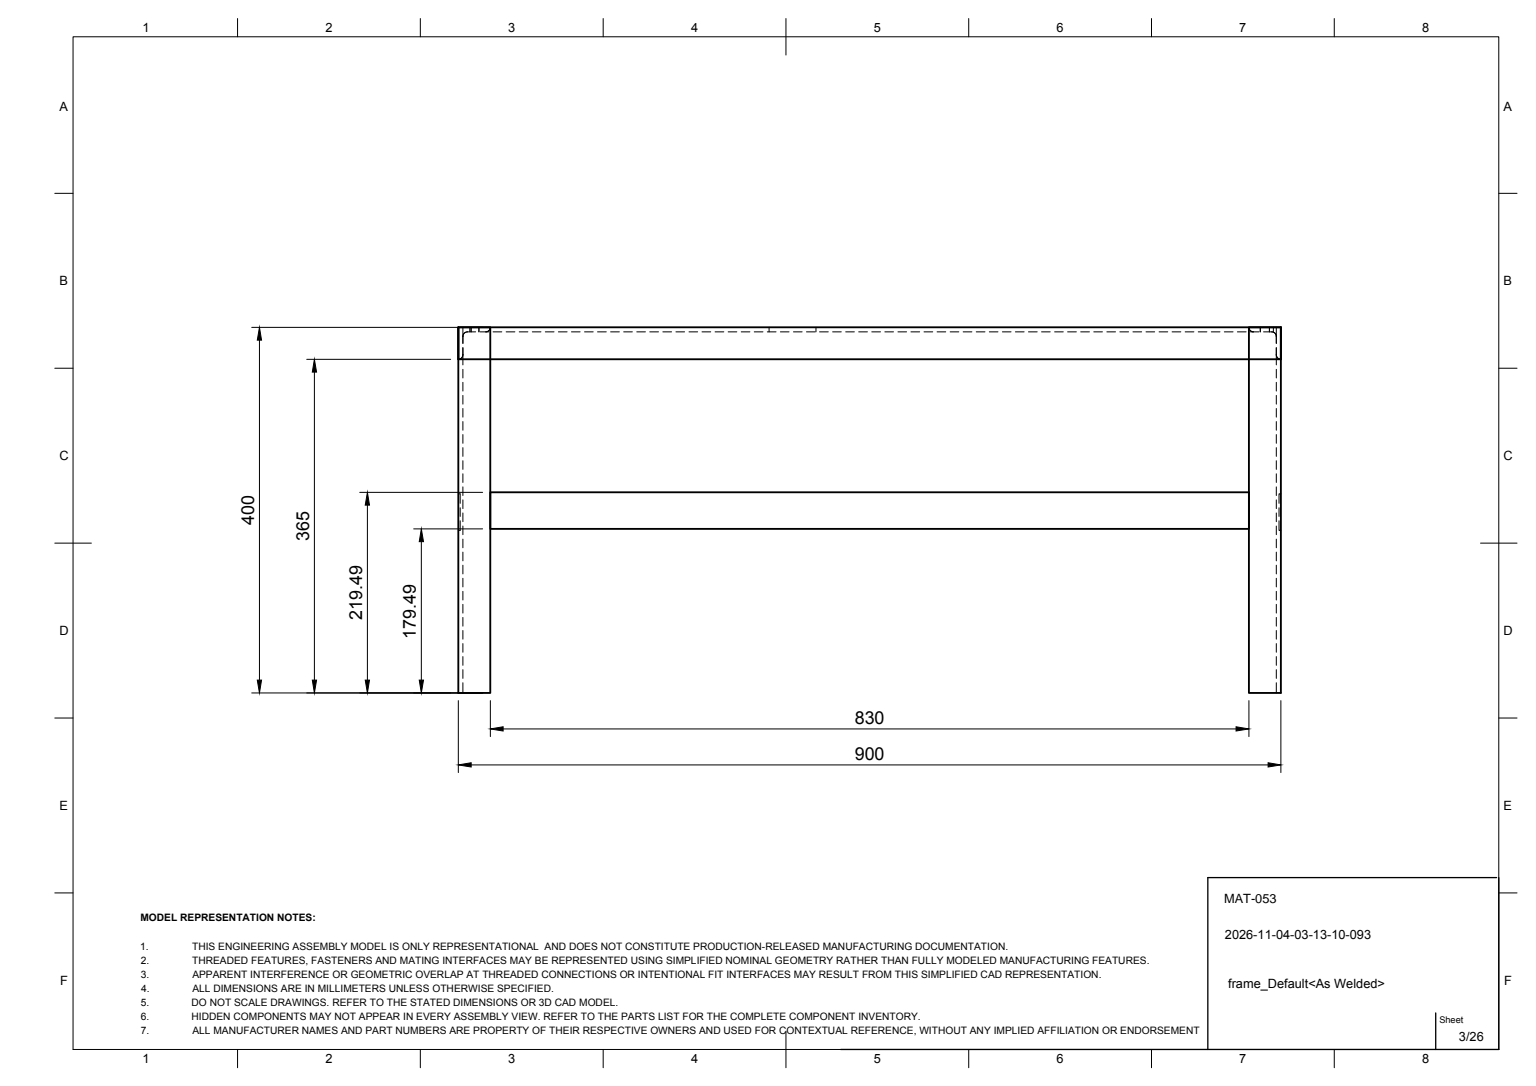
ISO-10303-21;
HEADER;
FILE_DESCRIPTION (('STEP AP214'),
    '1' );
FILE_NAME ('frame_Default<As Welded>.step',
    '2026-10-10T03:43:58',
    ( '' ),
    ( '' ),
    'SwSTEP 2.0',
    'SolidWorks 2026',
    '' );
FILE_SCHEMA (( 'AUTOMOTIVE_DESIGN' ));
ENDSEC;

DATA;
#18=ORIENTED_EDGE ( 'NONE', *, *, #43591, .T. ) ;
#28=DIRECTION ( 'NONE',  ( -1.000000000000000000, -1.850550996349095901E-16, -1.228197773518735191E-20 ) ) ;
#41=DIRECTION ( 'NONE',  ( -1.001915251000354105E-14, 1.000000000000000000, 5.551115123135531297E-17 ) ) ;
#49=CARTESIAN_POINT ( 'NONE',  ( 447.3372781065085633, 399.9999999999998863, 113.5502958579881891 ) ) ;
#135=VERTEX_POINT ( 'NONE', #41824 ) ;
#162=CARTESIAN_POINT ( 'NONE',  ( -444.4229916354184979, 394.6798985497181889, -128.9497041420121093 ) ) ;
#207=AXIS2_PLACEMENT_3D ( 'NONE', #62081, #45913, #12874 ) ;
#228=ORIENTED_EDGE ( 'NONE', *, *, #68309, .F. ) ;
#239=ORIENTED_EDGE ( 'NONE', *, *, #49975, .T. ) ;
#260=LINE ( 'NONE', #68864, #29041 ) ;
#261=VECTOR ( 'NONE', #60433, 1000.000000000000000 ) ;
#278=ORIENTED_EDGE ( 'NONE', *, *, #36224, .T. ) ;
#299=DIRECTION ( 'NONE',  ( 1.000000000000000000, 1.024558601614476894E-14, -9.899298618516476860E-15 ) ) ;
#301=VECTOR ( 'NONE', #7610, 1000.000000000000000 ) ;
#320=CARTESIAN_POINT ( 'NONE',  ( 442.3372781065083359, 370.0000000000043201, 108.5502958579838833 ) ) ;
#323=DIRECTION ( 'NONE',  ( 0.000000000000000000, 0.000000000000000000, -1.000000000000000000 ) ) ;
#329=FACE_OUTER_BOUND ( 'NONE', #61642, .T. ) ;
#352=DIRECTION ( 'NONE',  ( -0.7071067811865543451, -7.105427357601001070E-15, -0.7071067811865408004 ) ) ;
#366=VERTEX_POINT ( 'NONE', #38615 ) ;
#379=CYLINDRICAL_SURFACE ( 'NONE', #33876, 5.000000000000170530 ) ;
#403=AXIS2_PLACEMENT_3D ( 'NONE', #39353, #38653, #43213 ) ;
#416=CIRCLE ( 'NONE', #39744, 5.000000000000004441 ) ;
#423=AXIS2_PLACEMENT_3D ( 'NONE', #15656, #48667, #10364 ) ;
#492=CARTESIAN_POINT ( 'NONE',  ( -417.6627218934913230, 179.4906275429376308, 113.5502958579881749 ) ) ;
#493=DIRECTION ( 'NONE',  ( -2.921639538487254261E-16, -1.134144525784205431E-35, -1.000000000000000000 ) ) ;
#499=DIRECTION ( 'NONE',  ( 1.000000000000000000, 0.000000000000000000, 0.000000000000000000 ) ) ;
#500=ORIENTED_EDGE ( 'NONE', *, *, #39553, .F. ) ;
#508=DIRECTION ( 'NONE',  ( 1.000000000000000000, 0.000000000000000000, 0.000000000000000000 ) ) ;
#534=EDGE_CURVE ( 'NONE', #34523, #68707, #2552, .T. ) ;
#537=ORIENTED_EDGE ( 'NONE', *, *, #20232, .T. ) ;
#540=CARTESIAN_POINT ( 'NONE',  ( -442.6627218934913230, 1.665334536937734811E-13, 108.5502958579881749 ) ) ;
#568=VECTOR ( 'NONE', #4706, 1000.000000000000000 ) ;
#572=AXIS2_PLACEMENT_3D ( 'NONE', #9018, #25882, #35396 ) ;
#585=CARTESIAN_POINT ( 'NONE',  ( -422.6627218934914936, 399.9999999999998863, -141.4497041420118535 ) ) ;
#595=CARTESIAN_POINT ( 'NONE',  ( 107.3013380801408800, 395.0000000000065938, -128.9497041420121093 ) ) ;
#640=ADVANCED_FACE ( 'NONE', ( #57916 ), #9734, .T. ) ;
#646=CARTESIAN_POINT ( 'NONE',  ( 447.3372781065089612, 365.0000000000064233, -146.4497041420121377 ) ) ;
#648=ORIENTED_EDGE ( 'NONE', *, *, #3366, .T. ) ;
#665=FACE_OUTER_BOUND ( 'NONE', #60065, .T. ) ;
#678=CARTESIAN_POINT ( 'NONE',  ( 414.4083459183740388, 395.0000000000000568, -113.5207719538772579 ) ) ;
#699=CARTESIAN_POINT ( 'NONE',  ( 447.3372781065085633, 400.0000000000000568, -116.4497041420118393 ) ) ;
#723=CARTESIAN_POINT ( 'NONE',  ( -442.6627218934912662, 394.9999999999998295, 113.5502958579881465 ) ) ;
#726=ORIENTED_EDGE ( 'NONE', *, *, #5061, .T. ) ;
#732=CARTESIAN_POINT ( 'NONE',  ( -445.5916540816263591, 395.0000000000064801, -139.3786363301466906 ) ) ;
#742=ORIENTED_EDGE ( 'NONE', *, *, #24252, .T. ) ;
#756=AXIS2_PLACEMENT_3D ( 'NONE', #20145, #23779, #63754 ) ;
#768=ADVANCED_FACE ( 'NONE', ( #22611 ), #7498, .F. ) ;
#788=EDGE_CURVE ( 'NONE', #34907, #36914, #33986, .T. ) ;
#795=CARTESIAN_POINT ( 'NONE',  ( 412.3372781065085633, 219.4906275429376308, 113.5502958579881749 ) ) ;
#803=DIRECTION ( 'NONE',  ( -0.7071067811865405783, -7.105427357601001070E-15, 0.7071067811865545671 ) ) ;
#804=ORIENTED_EDGE ( 'NONE', *, *, #57601, .F. ) ;
#807=LINE ( 'NONE', #22262, #23012 ) ;
#810=ORIENTED_EDGE ( 'NONE', *, *, #68485, .F. ) ;
#817=EDGE_CURVE ( 'NONE', #39831, #41874, #11117, .T. ) ;
#829=ORIENTED_EDGE ( 'NONE', *, *, #20982, .F. ) ;
#869=CARTESIAN_POINT ( 'NONE',  ( -444.2280788262714282, 394.7493581867591388, -130.3782898954363532 ) ) ;
#876=EDGE_CURVE ( 'NONE', #55579, #9108, #39602, .T. ) ;
#907=AXIS2_PLACEMENT_3D ( 'NONE', #46556, #43247, #32374 ) ;
#910=VERTEX_POINT ( 'NONE', #6888 ) ;
#929=DIRECTION ( 'NONE',  ( 1.110223024625156540E-16, 1.358505038629840220E-33, 1.000000000000000000 ) ) ;
#957=FACE_OUTER_BOUND ( 'NONE', #48813, .T. ) ;
#966=DIRECTION ( 'NONE',  ( -1.000000000000000000, 0.000000000000000000, 0.000000000000000000 ) ) ;
#979=ORIENTED_EDGE ( 'NONE', *, *, #14468, .F. ) ;
#983=LINE ( 'NONE', #36278, #21334 ) ;
#1010=FACE_OUTER_BOUND ( 'NONE', #37761, .T. ) ;
#1019=DIRECTION ( 'NONE',  ( -1.000000000000000000, 0.000000000000000000, 0.000000000000000000 ) ) ;
#1062=FACE_OUTER_BOUND ( 'NONE', #64312, .T. ) ;
#1077=ORIENTED_EDGE ( 'NONE', *, *, #16773, .T. ) ;
#1078=CARTESIAN_POINT ( 'NONE',  ( -447.6627218934918346, 392.9289321881408910, -141.4497041420121661 ) ) ;
#1084=CYLINDRICAL_SURFACE ( 'NONE', #16978, 5.000000000000004441 ) ;
#1107=CARTESIAN_POINT ( 'NONE',  ( -443.8115333961470128, 394.8687311169578606, 93.62756966056487329 ) ) ;
#1126=LINE ( 'NONE', #65145, #9413 ) ;
#1128=DIRECTION ( 'NONE',  ( -1.000000000000000000, 1.232595164407830946E-32, 7.703719777548943412E-34 ) ) ;
#1133=CARTESIAN_POINT ( 'NONE',  ( -447.6627218934914367, 399.9999999999998863, -136.4497041420118251 ) ) ;
#1158=AXIS2_PLACEMENT_3D ( 'NONE', #24010, #19073, #25057 ) ;
#1160=DIRECTION ( 'NONE',  ( 1.232595164407830946E-32, 1.000000000000000000, 3.469446951953615421E-17 ) ) ;
#1222=CARTESIAN_POINT ( 'NONE',  ( 2.337278106504167230, 395.0000000000000000, -341.4497041420117966 ) ) ;
#1242=VECTOR ( 'NONE', #52232, 1000.000000000000000 ) ;
#1247=ORIENTED_EDGE ( 'NONE', *, *, #46850, .F. ) ;
#1264=DIRECTION ( 'NONE',  ( -3.081487911019579554E-32, -1.000000000000000000, -3.469446951953612956E-17 ) ) ;
#1275=LINE ( 'NONE', #22730, #301 ) ;
#1299=ORIENTED_EDGE ( 'NONE', *, *, #69235, .F. ) ;
#1342=CARTESIAN_POINT ( 'NONE',  ( 112.3013380801408658, 400.0000000000066507, -123.9497041420121235 ) ) ;
#1352=EDGE_CURVE ( 'NONE', #21613, #62663, #64860, .T. ) ;
#1391=ORIENTED_EDGE ( 'NONE', *, *, #21130, .F. ) ;
#1405=CARTESIAN_POINT ( 'NONE',  ( 442.3372781065085633, 399.9999999999998863, 103.5502958579881891 ) ) ;
#1409=ADVANCED_FACE ( 'NONE', ( #62002 ), #51117, .T. ) ;
#1411=EDGE_CURVE ( 'NONE', #51862, #23473, #29508, .T. ) ;
#1422=VECTOR ( 'NONE', #58262, 1000.000000000000000 ) ;
#1465=ORIENTED_EDGE ( 'NONE', *, *, #37162, .F. ) ;
#1521=VECTOR ( 'NONE', #55884, 1000.000000000000000 ) ;
#1538=VECTOR ( 'NONE', #21960, 1000.000000000000000 ) ;
#1541=CARTESIAN_POINT ( 'NONE',  ( -422.6627218934913230, 399.9999999999997726, 108.5502958579881891 ) ) ;
#1552=UNCERTAINTY_MEASURE_WITH_UNIT (LENGTH_MEASURE( 1.000000000000000082E-05 ), #45317, 'distance_accuracy_value', 'NONE');
#1580=VERTEX_POINT ( 'NONE', #18236 ) ;
#1591=LINE ( 'NONE', #17777, #28115 ) ;
#1592=LINE ( 'NONE', #44135, #22665 ) ;
#1640=DIRECTION ( 'NONE',  ( 1.850371928290090422E-16, -1.000000000000000000, -1.110223024625156171E-16 ) ) ;
#1652=EDGE_CURVE ( 'NONE', #46890, #13975, #15383, .T. ) ;
#1660=ORIENTED_EDGE ( 'NONE', *, *, #34022, .F. ) ;
#1666=EDGE_CURVE ( 'NONE', #1887, #55194, #16064, .T. ) ;
#1687=ADVANCED_FACE ( 'NONE', ( #31557 ), #48747, .F. ) ;
#1736=CARTESIAN_POINT ( 'NONE',  ( -20.16272189348855903, 400.0000000000064801, 321.0502958579853043 ) ) ;
#1748=DIRECTION ( 'NONE',  ( 0.000000000000000000, -1.000000000000000000, 0.000000000000000000 ) ) ;
#1776=CIRCLE ( 'NONE', #53407, 5.000000000000170530 ) ;
#1784=VERTEX_POINT ( 'NONE', #38561 ) ;
#1786=EDGE_CURVE ( 'NONE', #2896, #55220, #18505, .T. ) ;
#1787=CARTESIAN_POINT ( 'NONE',  ( -447.6627218934913230, 399.9999999999997726, 83.55029585798818914 ) ) ;
#1788=AXIS2_PLACEMENT_3D ( 'NONE', #24721, #40533, #2565 ) ;
#1808=FACE_OUTER_BOUND ( 'NONE', #63947, .T. ) ;
#1827=CARTESIAN_POINT ( 'NONE',  ( 445.3372781065085633, 177.8591479523844612, -111.4497041420119388 ) ) ;
#1838=VECTOR ( 'NONE', #46198, 1000.000000000000000 ) ;
#1849=AXIS2_PLACEMENT_3D ( 'NONE', #48486, #323, #32687 ) ;
#1868=ORIENTED_EDGE ( 'NONE', *, *, #4757, .T. ) ;
#1882=CARTESIAN_POINT ( 'NONE',  ( 447.3372781065085633, 217.8591479523844612, -111.4497041420119388 ) ) ;
#1887=VERTEX_POINT ( 'NONE', #41685 ) ;
#1891=FACE_OUTER_BOUND ( 'NONE', #33481, .T. ) ;
#1918=CARTESIAN_POINT ( 'NONE',  ( 112.3013380801408658, 388.0000000000065938, -123.9497041420121235 ) ) ;
#1981=ORIENTED_EDGE ( 'NONE', *, *, #63831, .F. ) ;
#1996=EDGE_CURVE ( 'NONE', #60543, #5635, #11609, .T. ) ;
#2025=FACE_OUTER_BOUND ( 'NONE', #12896, .T. ) ;
#2053=EDGE_CURVE ( 'NONE', #43634, #38637, #20566, .T. ) ;
#2108=CARTESIAN_POINT ( 'NONE',  ( 424.8372781065087906, 400.0000000000067075, -123.9497041420121235 ) ) ;
#2130=( GEOMETRIC_REPRESENTATION_CONTEXT ( 3 ) GLOBAL_UNCERTAINTY_ASSIGNED_CONTEXT ( ( #8581 ) ) GLOBAL_UNIT_ASSIGNED_CONTEXT ( ( #28794, #2407, #61144 ) ) REPRESENTATION_CONTEXT ( 'NONE', 'WORKASPACE' ) );
#2145=EDGE_LOOP ( 'NONE', ( #5278, #8405, #51535 ) ) ;
#2147=CARTESIAN_POINT ( 'NONE',  ( -442.6627218934916641, 394.9999999999954525, 103.5502958579924808 ) ) ;
#2180=ORIENTED_EDGE ( 'NONE', *, *, #21990, .T. ) ;
#2250=AXIS2_PLACEMENT_3D ( 'NONE', #44344, #38734, #56292 ) ;
#2260=DIRECTION ( 'NONE',  ( 0.000000000000000000, 1.000000000000000000, 0.000000000000000000 ) ) ;
#2295=DIRECTION ( 'NONE',  ( -1.000000000000000000, 0.000000000000000000, 0.000000000000000000 ) ) ;
#2296=CARTESIAN_POINT ( 'NONE',  ( 445.3372781065086201, 177.8591479523844612, 78.55029585798806124 ) ) ;
#2306=EDGE_CURVE ( 'NONE', #4870, #42101, #55269, .T. ) ;
#2311=ORIENTED_EDGE ( 'NONE', *, *, #31125, .T. ) ;
#2325=ORIENTED_EDGE ( 'NONE', *, *, #51865, .F. ) ;
#2331=PLANE ( 'NONE',  #41598 ) ;
#2335=ORIENTED_EDGE ( 'NONE', *, *, #23615, .F. ) ;
#2342=LINE ( 'NONE', #66717, #52285 ) ;
#2350=SHAPE_REPRESENTATION_RELATIONSHIP ( 'NONE' , 'NONE' ,  #2894, #64275 ) ;
#2405=STYLED_ITEM ( 'NONE', ( #35553 ), #16744 ) ;
#2406=DIRECTION ( 'NONE',  ( -4.270088556250601699E-16, -0.000000000000000000, -1.000000000000000000 ) ) ;
#2407=( NAMED_UNIT ( * ) PLANE_ANGLE_UNIT ( ) SI_UNIT ( $, .RADIAN. ) );
#2464=EDGE_LOOP ( 'NONE', ( #43968, #36978, #53446, #55906, #66488, #18902, #35917 ) ) ;
#2487=ADVANCED_FACE ( 'NONE', ( #5266 ), #48156, .T. ) ;
#2503=DIRECTION ( 'NONE',  ( 1.387778780781446169E-16, -1.000000000000000000, -3.469446951953615421E-17 ) ) ;
#2532=CARTESIAN_POINT ( 'NONE',  ( -417.6627218934913799, 399.9999999999998295, -111.4497041420118251 ) ) ;
#2536=CARTESIAN_POINT ( 'NONE',  ( -444.4229916354184979, 394.6798985497181320, 96.05029585798874336 ) ) ;
#2552=CIRCLE ( 'NONE', #39606, 5.000000000000004441 ) ;
#2565=DIRECTION ( 'NONE',  ( 1.000000000000000000, -9.109522253334613014E-16, 0.000000000000000000 ) ) ;
#2568=EDGE_CURVE ( 'NONE', #37758, #24336, #57705, .T. ) ;
#2583=ORIENTED_EDGE ( 'NONE', *, *, #50107, .F. ) ;
#2595=VECTOR ( 'NONE', #6924, 1000.000000000000000 ) ;
#2601=AXIS2_PLACEMENT_3D ( 'NONE', #24393, #62712, #45834 ) ;
#2604=ORIENTED_EDGE ( 'NONE', *, *, #10155, .T. ) ;
#2622=DIRECTION ( 'NONE',  ( 1.000000000000000000, 0.000000000000000000, 0.000000000000000000 ) ) ;
#2624=CARTESIAN_POINT ( 'NONE',  ( -452.6627218934912662, 364.9999999999998863, 113.5502958579877912 ) ) ;
#2681=LINE ( 'NONE', #55439, #22046 ) ;
#2713=EDGE_LOOP ( 'NONE', ( #26660, #62305, #27434, #31457 ) ) ;
#2752=FACE_OUTER_BOUND ( 'NONE', #52532, .T. ) ;
#2761=( NAMED_UNIT ( * ) PLANE_ANGLE_UNIT ( ) SI_UNIT ( $, .RADIAN. ) );
#2765=CARTESIAN_POINT ( 'NONE',  ( 112.3013380801407095, 388.0000000000077307, 91.05029585798746439 ) ) ;
#2771=CARTESIAN_POINT ( 'NONE',  ( -452.6627218934912094, 399.9999999999998295, 113.5502958579882602 ) ) ;
#2791=CARTESIAN_POINT ( 'NONE',  ( -452.6627218934913230, 399.9999999999997726, 78.55029585798818914 ) ) ;
#2833=PLANE ( 'NONE',  #68014 ) ;
#2834=VECTOR ( 'NONE', #1264, 1000.000000000000000 ) ;
#2838=CARTESIAN_POINT ( 'NONE',  ( 412.3372781065085633, 219.4906275429376308, 111.5502958579881749 ) ) ;
#2857=VERTEX_POINT ( 'NONE', #66811 ) ;
#2884=EDGE_CURVE ( 'NONE', #36808, #910, #34790, .T. ) ;
#2891=VECTOR ( 'NONE', #10003, 1000.000000000000000 ) ;
#2894=SHAPE_REPRESENTATION ( 'frame_Default<As Welded>', ( #66832 ), #12890 ) ;
#2896=VERTEX_POINT ( 'NONE', #68432 ) ;
#2914=ORIENTED_EDGE ( 'NONE', *, *, #9847, .T. ) ;
#2925=CARTESIAN_POINT ( 'NONE',  ( -450.6627218934913230, 217.8591479523843475, 78.55029585798814651 ) ) ;
#2948=EDGE_CURVE ( 'NONE', #44967, #17356, #65568, .T. ) ;
#2953=EDGE_CURVE ( 'NONE', #6937, #46890, #35233, .T. ) ;
#2955=EDGE_CURVE ( 'NONE', #36796, #51074, #58217, .T. ) ;
#2956=CARTESIAN_POINT ( 'NONE',  ( -439.4229916354183274, 400.0000000000064801, 96.05029585798874336 ) ) ;
#2958=CARTESIAN_POINT ( 'NONE',  ( 437.3372781065085633, 390.0000000000001137, -146.4497041420117966 ) ) ;
#2979=DIRECTION ( 'NONE',  ( -1.387778780781445922E-16, 1.000000000000000000, 1.232595164407830946E-32 ) ) ;
#2980=DIRECTION ( 'NONE',  ( 9.729495617646301779E-15, -5.551115123125782702E-17, 1.000000000000000000 ) ) ;
#2982=VECTOR ( 'NONE', #47038, 1000.000000000000000 ) ;
#2983=ORIENTED_EDGE ( 'NONE', *, *, #34114, .F. ) ;
#2985=DIRECTION ( 'NONE',  ( -1.000000000000000000, 0.000000000000000000, 0.000000000000000000 ) ) ;
#3011=DIRECTION ( 'NONE',  ( -1.000000000000000000, 0.000000000000000000, 0.000000000000000000 ) ) ;
#3038=AXIS2_PLACEMENT_3D ( 'NONE', #5533, #54754, #23111 ) ;
#3044=EDGE_LOOP ( 'NONE', ( #2914, #25695, #29990, #1660 ) ) ;
#3057=PLANE ( 'NONE',  #30957 ) ;
#3091=AXIS2_PLACEMENT_3D ( 'NONE', #61680, #34958, #66297 ) ;
#3096=EDGE_CURVE ( 'NONE', #32147, #11742, #65456, .T. ) ;
#3100=ORIENTED_EDGE ( 'NONE', *, *, #817, .T. ) ;
#3113=VERTEX_POINT ( 'NONE', #34963 ) ;
#3116=ADVANCED_FACE ( 'NONE', ( #51138 ), #14198, .T. ) ;
#3120=CARTESIAN_POINT ( 'NONE',  ( -452.6627218934918346, 365.0000000000064233, -146.4497041420121377 ) ) ;
#3122=( NAMED_UNIT ( * ) PLANE_ANGLE_UNIT ( ) SI_UNIT ( $, .RADIAN. ) );
#3151=ADVANCED_FACE ( 'NONE', ( #51491 ), #25107, .T. ) ;
#3161=VERTEX_POINT ( 'NONE', #9956 ) ;
#3167=ORIENTED_EDGE ( 'NONE', *, *, #33592, .T. ) ;
#3207=CARTESIAN_POINT ( 'NONE',  ( 442.3372781065085633, 400.0000000000000568, -116.4497041420118393 ) ) ;
#3224=CARTESIAN_POINT ( 'NONE',  ( 437.3372781065085633, 399.9999999999998863, 103.5502958579881891 ) ) ;
#3237=AXIS2_PLACEMENT_3D ( 'NONE', #6631, #26704, #65382 ) ;
#3240=CARTESIAN_POINT ( 'NONE',  ( 417.3372781065086770, 0.000000000000000000, 108.5502958579881891 ) ) ;
#3251=CARTESIAN_POINT ( 'NONE',  ( -417.6627218934913230, 219.4906275429376308, -146.4497041420118819 ) ) ;
#3257=EDGE_CURVE ( 'NONE', #19058, #41538, #58468, .T. ) ;
#3264=EDGE_LOOP ( 'NONE', ( #28641, #52255, #19541, #43229, #54328, #3932, #7134, #33574, #55209, #62511, #15106, #27197 ) ) ;
#3289=LINE ( 'NONE', #24747, #33740 ) ;
#3298=CARTESIAN_POINT ( 'NONE',  ( 437.3372781065085633, 395.0000000000001137, -146.4497041420117966 ) ) ;
#3304=CARTESIAN_POINT ( 'NONE',  ( 412.3372781065085633, 219.4906275429376308, 113.5502958579881749 ) ) ;
#3316=FACE_OUTER_BOUND ( 'NONE', #58462, .T. ) ;
#3319=ORIENTED_EDGE ( 'NONE', *, *, #44714, .T. ) ;
#3338=DIRECTION ( 'NONE',  ( 0.000000000000000000, 6.123233995736761105E-17, -1.000000000000000000 ) ) ;
#3362=AXIS2_PLACEMENT_3D ( 'NONE', #53763, #27037, #48468 ) ;
#3366=EDGE_CURVE ( 'NONE', #60705, #17566, #50001, .T. ) ;
#3371=VERTEX_POINT ( 'NONE', #54575 ) ;
#3393=CARTESIAN_POINT ( 'NONE',  ( -447.6627218934919483, 370.0000000000056275, -141.4497041420121661 ) ) ;
#3394=CARTESIAN_POINT ( 'NONE',  ( 14.83727810650406731, 400.0000000000001137, -353.9497041420119672 ) ) ;
#3400=ORIENTED_EDGE ( 'NONE', *, *, #22879, .F. ) ;
#3414=ORIENTED_EDGE ( 'NONE', *, *, #12766, .T. ) ;
#3424=EDGE_LOOP ( 'NONE', ( #40584, #35783, #60824, #8916 ) ) ;
#3438=PLANE ( 'NONE',  #44136 ) ;
#3450=ORIENTED_EDGE ( 'NONE', *, *, #23507, .T. ) ;
#3458=CARTESIAN_POINT ( 'NONE',  ( -452.6627218934913799, 364.9999999999998295, -146.4497041420117966 ) ) ;
#3460=AXIS2_PLACEMENT_3D ( 'NONE', #7707, #40739, #29155 ) ;
#3481=CARTESIAN_POINT ( 'NONE',  ( 447.3372781065086201, 0.000000000000000000, 83.55029585798817493 ) ) ;
#3487=DIRECTION ( 'NONE',  ( 1.387778780781445429E-16, -1.000000000000000000, -3.081487911019577365E-33 ) ) ;
#3490=VECTOR ( 'NONE', #9251, 1000.000000000000114 ) ;
#3534=SURFACE_SIDE_STYLE ('',( #42208 ) ) ;
#3547=VECTOR ( 'NONE', #40734, 1000.000000000000000 ) ;
#3549=DIRECTION ( 'NONE',  ( 0.7071067811865476838, 1.110223024625156294E-16, 0.7071067811865474617 ) ) ;
#3582=ORIENTED_EDGE ( 'NONE', *, *, #15343, .F. ) ;
#3586=AXIS2_PLACEMENT_3D ( 'NONE', #12327, #33447, #27444 ) ;
#3590=VECTOR ( 'NONE', #42220, 1000.000000000000000 ) ;
#3631=DIRECTION ( 'NONE',  ( 0.7071067811865474617, -5.551115123125781716E-16, 0.7071067811865475727 ) ) ;
#3632=ADVANCED_FACE ( 'NONE', ( #23511 ), #48674, .T. ) ;
#3644=EDGE_CURVE ( 'NONE', #21636, #60543, #50981, .T. ) ;
#3649=AXIS2_PLACEMENT_3D ( 'NONE', #4128, #13639, #40372 ) ;
#3651=LINE ( 'NONE', #53889, #16378 ) ;
#3702=CARTESIAN_POINT ( 'NONE',  ( 447.3372781065085633, 400.0000000000000568, -146.4497041420118251 ) ) ;
#3703=CARTESIAN_POINT ( 'NONE',  ( 412.3372781065082791, 400.0000000000040927, 78.55029585798418168 ) ) ;
#3716=ORIENTED_EDGE ( 'NONE', *, *, #64221, .T. ) ;
#3753=ADVANCED_FACE ( 'NONE', ( #59941 ), #6837, .T. ) ;
#3759=DIRECTION ( 'NONE',  ( 6.405132834375901070E-16, -1.000000000000000000, -6.405132834375902056E-16 ) ) ;
#3784=ADVANCED_FACE ( 'NONE', ( #7893 ), #49385, .T. ) ;
#3804=CARTESIAN_POINT ( 'NONE',  ( -452.6627218934914367, 399.9999999999998863, -146.4497041420118251 ) ) ;
#3849=ORIENTED_EDGE ( 'NONE', *, *, #26324, .F. ) ;
#3854=EDGE_LOOP ( 'NONE', ( #26584, #28103, #17107, #64079, #38779, #9643, #4054 ) ) ;
#3867=EDGE_LOOP ( 'NONE', ( #36108, #28405, #537, #61706 ) ) ;
#3892=DIRECTION ( 'NONE',  ( 0.000000000000000000, -6.123233995736762338E-17, 1.000000000000000000 ) ) ;
#3904=LINE ( 'NONE', #29250, #45362 ) ;
#3929=ORIENTED_EDGE ( 'NONE', *, *, #39789, .T. ) ;
#3932=ORIENTED_EDGE ( 'NONE', *, *, #3096, .T. ) ;
#3959=EDGE_CURVE ( 'NONE', #38702, #53656, #25115, .T. ) ;
#3963=ORIENTED_EDGE ( 'NONE', *, *, #8078, .F. ) ;
#4033=ORIENTED_EDGE ( 'NONE', *, *, #59864, .T. ) ;
#4050=ADVANCED_FACE ( 'NONE', ( #31754 ), #69386, .T. ) ;
#4054=ORIENTED_EDGE ( 'NONE', *, *, #64477, .F. ) ;
#4055=DIRECTION ( 'NONE',  ( -1.000000000000000000, 1.540743955509788682E-33, 1.110223024625156540E-16 ) ) ;
#4098=ORIENTED_EDGE ( 'NONE', *, *, #66400, .T. ) ;
#4118=EDGE_LOOP ( 'NONE', ( #27509, #50059, #51468, #64476, #63468, #11482, #54903 ) ) ;
#4128=CARTESIAN_POINT ( 'NONE',  ( -422.6627218934914367, 0.000000000000000000, -146.4497041420118251 ) ) ;
#4132=ADVANCED_FACE ( 'NONE', ( #15922 ), #15236, .T. ) ;
#4156=CARTESIAN_POINT ( 'NONE',  ( -449.7337897053568554, 364.9999999999998295, -143.5207719538772722 ) ) ;
#4159=ORIENTED_EDGE ( 'NONE', *, *, #52250, .F. ) ;
#4203=CARTESIAN_POINT ( 'NONE',  ( 437.3372781065085633, 394.9999999999999432, 91.05029585798857283 ) ) ;
#4214=CARTESIAN_POINT ( 'NONE',  ( 412.3372781065085633, 219.4906275429376308, -144.4497041420117682 ) ) ;
#4215=VERTEX_POINT ( 'NONE', #29594 ) ;
#4254=DIRECTION ( 'NONE',  ( 1.387778780781445922E-16, -1.000000000000000000, -1.232595164407830946E-32 ) ) ;
#4271=EDGE_LOOP ( 'NONE', ( #40131, #56927, #23005, #48343 ) ) ;
#4293=VECTOR ( 'NONE', #68342, 1000.000000000000000 ) ;
#4319=CARTESIAN_POINT ( 'NONE',  ( 445.3372781065086201, 177.8591479523844612, 78.55029585798806124 ) ) ;
#4339=( GEOMETRIC_REPRESENTATION_CONTEXT ( 3 ) GLOBAL_UNCERTAINTY_ASSIGNED_CONTEXT ( ( #9258 ) ) GLOBAL_UNIT_ASSIGNED_CONTEXT ( ( #38027, #66523, #46082 ) ) REPRESENTATION_CONTEXT ( 'NONE', 'WORKASPACE' ) );
#4340=DIRECTION ( 'NONE',  ( -4.946224812893509176E-48, 1.000000000000000000, 3.697785493223491743E-32 ) ) ;
#4348=EDGE_LOOP ( 'NONE', ( #4033, #62830, #17819, #64317 ) ) ;
#4384=AXIS2_PLACEMENT_3D ( 'NONE', #3481, #29873, #67509 ) ;
#4395=CARTESIAN_POINT ( 'NONE',  ( -417.6627218934913230, 219.4906275429376308, 111.5502958579881749 ) ) ;
#4400=DIRECTION ( 'NONE',  ( -3.946780934433987212E-15, -1.000000000000000000, 5.551115123125782702E-17 ) ) ;
#4404=VERTEX_POINT ( 'NONE', #67182 ) ;
#4450=DIRECTION ( 'NONE',  ( -0.7071067811865543451, -7.105427357601001070E-15, -0.7071067811865408004 ) ) ;
#4458=ADVANCED_FACE ( 'NONE', ( #43861 ), #27341, .T. ) ;
#4492=CARTESIAN_POINT ( 'NONE',  ( 437.3372781065086201, 0.000000000000000000, -141.4497041420118251 ) ) ;
#4507=ORIENTED_EDGE ( 'NONE', *, *, #67988, .F. ) ;
#4515=DIRECTION ( 'NONE',  ( 0.7071067811865475727, 0.000000000000000000, 0.7071067811865474617 ) ) ;
#4564=DIRECTION ( 'NONE',  ( 1.000000000000000000, 3.697785493223491743E-32, 0.000000000000000000 ) ) ;
#4617=EDGE_CURVE ( 'NONE', #55210, #15602, #36710, .T. ) ;
#4632=LINE ( 'NONE', #15196, #49150 ) ;
#4649=SURFACE_STYLE_USAGE ( .BOTH. , #58450 ) ;
#4650=PLANE ( 'NONE',  #24544 ) ;
#4654=EDGE_CURVE ( 'NONE', #23082, #15354, #60817, .T. ) ;
#4675=VERTEX_POINT ( 'NONE', #37729 ) ;
#4691=COLOUR_RGB ( '',0.7921568627450980005, 0.8196078431372548767, 0.9333333333333333481 ) ;
#4706=DIRECTION ( 'NONE',  ( 0.000000000000000000, -1.000000000000000000, 1.479221584281239571E-31 ) ) ;
#4708=ORIENTED_EDGE ( 'NONE', *, *, #14752, .F. ) ;
#4757=EDGE_CURVE ( 'NONE', #38637, #41110, #62186, .T. ) ;
#4775=VERTEX_POINT ( 'NONE', #2536 ) ;
#4811=LINE ( 'NONE', #15720, #2982 ) ;
#4836=EDGE_LOOP ( 'NONE', ( #31185, #40353, #53092, #63097 ) ) ;
#4838=FILL_AREA_STYLE_COLOUR ( '', #64366 ) ;
#4870=VERTEX_POINT ( 'NONE', #26755 ) ;
#4877=ORIENTED_EDGE ( 'NONE', *, *, #51267, .T. ) ;
#4921=ORIENTED_EDGE ( 'NONE', *, *, #14230, .T. ) ;
#4953=EDGE_LOOP ( 'NONE', ( #54643, #42832, #50469, #17326 ) ) ;
#4963=ORIENTED_EDGE ( 'NONE', *, *, #67890, .F. ) ;
#4969=CARTESIAN_POINT ( 'NONE',  ( 429.8372781065087338, 388.0000000000065938, 91.05029585798857283 ) ) ;
#4971=CARTESIAN_POINT ( 'NONE',  ( 445.3372781065085633, 177.8591479523844612, -111.4497041420119388 ) ) ;
#4988=EDGE_LOOP ( 'NONE', ( #67374, #3849, #16908, #44677, #2325, #29922, #50568 ) ) ;
#5005=ORIENTED_EDGE ( 'NONE', *, *, #30906, .T. ) ;
#5020=VECTOR ( 'NONE', #68078, 1000.000000000000000 ) ;
#5023=CARTESIAN_POINT ( 'NONE',  ( -439.4229916354183842, 388.0000000000064801, -128.9497041420121093 ) ) ;
#5031=AXIS2_PLACEMENT_3D ( 'NONE', #48409, #43149, #64619 ) ;
#5050=EDGE_CURVE ( 'NONE', #55210, #28296, #17940, .T. ) ;
#5061=EDGE_CURVE ( 'NONE', #67779, #9014, #65792, .T. ) ;
#5064=DIRECTION ( 'NONE',  ( -1.000000000000000000, 0.000000000000000000, -1.110223024625156294E-16 ) ) ;
#5084=ORIENTED_EDGE ( 'NONE', *, *, #25971, .T. ) ;
#5101=DIRECTION ( 'NONE',  ( 1.000000000000000000, 1.001918829714556097E-14, -9.899279560275163638E-15 ) ) ;
#5103=CARTESIAN_POINT ( 'NONE',  ( -442.6627218934913799, 0.000000000000000000, -136.4497041420118251 ) ) ;
#5135=( BOUNDED_CURVE ( )  B_SPLINE_CURVE ( 3, ( #39750, #65803, #55574, #17599 ),
 .UNSPECIFIED., .F., .F. ) 
 B_SPLINE_CURVE_WITH_KNOTS ( ( 4, 4 ),
 ( 1.570796326794883679, 3.141592653589778461 ),
 .UNSPECIFIED. ) 
 CURVE ( )  GEOMETRIC_REPRESENTATION_ITEM ( )  RATIONAL_B_SPLINE_CURVE ( ( 1.000000000000000000, 0.8047378541243654926, 0.8047378541243654926, 1.000000000000000000 ) ) 
 REPRESENTATION_ITEM ( '' )  );
#5153=DIRECTION ( 'NONE',  ( -1.000000000000000000, 0.000000000000000000, 0.000000000000000000 ) ) ;
#5187=ORIENTED_EDGE ( 'NONE', *, *, #12766, .F. ) ;
#5225=DIRECTION ( 'NONE',  ( 1.387778780781445922E-16, -1.000000000000000000, 0.000000000000000000 ) ) ;
#5228=FACE_OUTER_BOUND ( 'NONE', #4118, .T. ) ;
#5234=EDGE_CURVE ( 'NONE', #25372, #38916, #8075, .T. ) ;
#5247=SURFACE_STYLE_USAGE ( .BOTH. , #43554 ) ;
#5266=FACE_OUTER_BOUND ( 'NONE', #39432, .T. ) ;
#5278=ORIENTED_EDGE ( 'NONE', *, *, #1996, .F. ) ;
#5286=AXIS2_PLACEMENT_3D ( 'NONE', #46791, #20396, #24661 ) ;
#5302=ADVANCED_FACE ( 'NONE', ( #29524 ), #29883, .T. ) ;
#5384=CARTESIAN_POINT ( 'NONE',  ( -417.6627218934913230, 179.4906275429376308, 111.5502958579881749 ) ) ;
#5412=DIRECTION ( 'NONE',  ( 1.000000000000000000, 1.850550996349095901E-16, 1.228197773518735191E-20 ) ) ;
#5416=DIRECTION ( 'NONE',  ( -0.7071067811865473507, 6.441404958702665783E-16, 0.7071067811865477948 ) ) ;
#5448=CARTESIAN_POINT ( 'NONE',  ( -442.6627218934913799, 394.9999999999998295, -132.7581352960343679 ) ) ;
#5476=STYLED_ITEM ( 'NONE', ( #48551 ), #63846 ) ;
#5480=EDGE_LOOP ( 'NONE', ( #45183, #46394, #64906, #1077 ) ) ;
#5511=VERTEX_POINT ( 'NONE', #34038 ) ;
#5513=ORIENTED_EDGE ( 'NONE', *, *, #56243, .F. ) ;
#5533=CARTESIAN_POINT ( 'NONE',  ( 412.3372781065085633, 179.4906275429376024, 111.5502958579881749 ) ) ;
#5545=EDGE_CURVE ( 'NONE', #17804, #45879, #49845, .T. ) ;
#5564=VERTEX_POINT ( 'NONE', #55478 ) ;
#5579=EDGE_LOOP ( 'NONE', ( #67998, #13822, #65351, #59763 ) ) ;
#5593=CARTESIAN_POINT ( 'NONE',  ( -447.6627218934913799, 370.0000000000002274, -141.4497041420117966 ) ) ;
#5596=CARTESIAN_POINT ( 'NONE',  ( -422.6627218934914936, 399.9999999999998863, -141.4497041420118535 ) ) ;
#5635=VERTEX_POINT ( 'NONE', #42417 ) ;
#5642=CARTESIAN_POINT ( 'NONE',  ( 429.8372781065087338, 400.0000000000067075, -123.9497041420121235 ) ) ;
#5661=FACE_OUTER_BOUND ( 'NONE', #23819, .T. ) ;
#5663=DIRECTION ( 'NONE',  ( -1.850169831522831466E-16, 1.000000000000000000, 1.110223024625156294E-16 ) ) ;
#5693=VECTOR ( 'NONE', #9339, 999.9999999999998863 ) ;
#5702=DIRECTION ( 'NONE',  ( -1.850169831522831466E-16, 1.000000000000000000, 1.110223024625156294E-16 ) ) ;
#5731=ORIENTED_EDGE ( 'NONE', *, *, #3644, .T. ) ;
#5774=CIRCLE ( 'NONE', #15927, 5.000000000000004441 ) ;
#5806=ORIENTED_EDGE ( 'NONE', *, *, #10304, .T. ) ;
#5816=CARTESIAN_POINT ( 'NONE',  ( -417.6627218934913230, 179.4906275429376308, 113.5502958579881749 ) ) ;
#5823=VECTOR ( 'NONE', #69312, 1000.000000000000000 ) ;
#5857=CARTESIAN_POINT ( 'NONE',  ( 412.3372781065085633, 179.4906275429376024, 113.5502958579881749 ) ) ;
#5872=ORIENTED_EDGE ( 'NONE', *, *, #30906, .F. ) ;
#5915=CARTESIAN_POINT ( 'NONE',  ( -450.6627218934913230, 217.8591479523843475, 78.55029585798814651 ) ) ;
#5935=LINE ( 'NONE', #43575, #29982 ) ;
#5952=EDGE_CURVE ( 'NONE', #6104, #67779, #27617, .T. ) ;
#5966=FACE_OUTER_BOUND ( 'NONE', #56010, .T. ) ;
#5979=CIRCLE ( 'NONE', #21708, 5.000000000000004441 ) ;
#5994=LINE ( 'NONE', #36987, #7817 ) ;
#6017=VERTEX_POINT ( 'NONE', #40958 ) ;
#6037=VECTOR ( 'NONE', #41872, 1000.000000000000000 ) ;
#6052=LINE ( 'NONE', #54591, #30147 ) ;
#6059=CARTESIAN_POINT ( 'NONE',  ( 442.3372781065085633, 369.9999999999999432, 108.5502958579885870 ) ) ;
#6087=CYLINDRICAL_SURFACE ( 'NONE', #32050, 5.000000000000004441 ) ;
#6104=VERTEX_POINT ( 'NONE', #65088 ) ;
#6117=FACE_OUTER_BOUND ( 'NONE', #68741, .T. ) ;
#6120=DIRECTION ( 'NONE',  ( -0.7071067811865474617, 9.422489238170280455E-15, 0.7071067811865475727 ) ) ;
#6124=DIRECTION ( 'NONE',  ( 4.314083075427411048E-32, 1.000000000000000000, 6.123233995736763571E-17 ) ) ;
#6146=PLANE ( 'NONE',  #6687 ) ;
#6187=VECTOR ( 'NONE', #64225, 1000.000000000000000 ) ;
#6215=DIRECTION ( 'NONE',  ( 1.387778780781446169E-16, -1.000000000000000000, -3.469446951953615421E-17 ) ) ;
#6247=CARTESIAN_POINT ( 'NONE',  ( 112.3013380801408658, 388.0000000000065938, -133.9497041420121377 ) ) ;
#6288=LINE ( 'NONE', #48826, #31905 ) ;
#6315=ORIENTED_EDGE ( 'NONE', *, *, #50891, .F. ) ;
#6342=DIRECTION ( 'NONE',  ( -4.270088556250601699E-16, -0.000000000000000000, -1.000000000000000000 ) ) ;
#6347=DIRECTION ( 'NONE',  ( -4.270088556250601699E-16, -0.000000000000000000, -1.000000000000000000 ) ) ;
#6360=ORIENTED_EDGE ( 'NONE', *, *, #47873, .F. ) ;
#6369=CARTESIAN_POINT ( 'NONE',  ( -450.6627218934913230, 177.8591479523843475, -111.4497041420117966 ) ) ;
#6379=VECTOR ( 'NONE', #25784, 1000.000000000000000 ) ;
#6427=EDGE_CURVE ( 'NONE', #50950, #65355, #5135, .T. ) ;
#6435=EDGE_CURVE ( 'NONE', #43624, #59231, #39062, .T. ) ;
#6436=VECTOR ( 'NONE', #45427, 1000.000000000000000 ) ;
#6470=LINE ( 'NONE', #27563, #69136 ) ;
#6501=EDGE_CURVE ( 'NONE', #6937, #3371, #65968, .T. ) ;
#6503=LINE ( 'NONE', #1222, #13627 ) ;
#6507=CARTESIAN_POINT ( 'NONE',  ( -417.6627218934913230, 179.4906275429376308, 111.5502958579881749 ) ) ;
#6563=ORIENTED_EDGE ( 'NONE', *, *, #33056, .F. ) ;
#6579=FACE_OUTER_BOUND ( 'NONE', #7176, .T. ) ;
#6599=CARTESIAN_POINT ( 'NONE',  ( -444.4229916354184979, 400.0000000000064801, 96.05029585798874336 ) ) ;
#6630=CARTESIAN_POINT ( 'NONE',  ( 447.3372781065085633, 399.9999999999998863, 113.5502958579882034 ) ) ;
#6631=CARTESIAN_POINT ( 'NONE',  ( 112.3013380801407521, 388.0000000000077307, 96.05029585798746439 ) ) ;
#6659=EDGE_CURVE ( 'NONE', #54476, #2896, #67975, .T. ) ;
#6662=ADVANCED_FACE ( 'NONE', ( #62473 ), #14963, .T. ) ;
#6683=CARTESIAN_POINT ( 'NONE',  ( 433.3728120124415568, 400.0000000000067075, -132.4852380479448755 ) ) ;
#6687=AXIS2_PLACEMENT_3D ( 'NONE', #17042, #33947, #27958 ) ;
#6733=AXIS2_PLACEMENT_3D ( 'NONE', #63708, #15519, #68627 ) ;
#6746=AXIS2_PLACEMENT_3D ( 'NONE', #10254, #41, #48555 ) ;
#6783=DIRECTION ( 'NONE',  ( -1.000000000000000000, -1.850474763383843014E-16, 1.697708136181793677E-16 ) ) ;
#6798=EDGE_CURVE ( 'NONE', #1784, #51862, #11794, .T. ) ;
#6807=EDGE_LOOP ( 'NONE', ( #20423, #68819, #14156, #34926 ) ) ;
#6822=EDGE_CURVE ( 'NONE', #42101, #40754, #62676, .T. ) ;
#6837=PLANE ( 'NONE',  #43037 ) ;
#6848=EDGE_CURVE ( 'NONE', #34711, #44967, #33965, .T. ) ;
#6852=AXIS2_PLACEMENT_3D ( 'NONE', #35683, #2980, #8249 ) ;
#6853=ORIENTED_EDGE ( 'NONE', *, *, #17658, .T. ) ;
#6857=VECTOR ( 'NONE', #3338, 1000.000000000000000 ) ;
#6888=CARTESIAN_POINT ( 'NONE',  ( 50.98853755884156413, 400.0000000000065938, -133.9497041420122798 ) ) ;
#6890=ORIENTED_EDGE ( 'NONE', *, *, #63616, .F. ) ;
#6891=VECTOR ( 'NONE', #43073, 1000.000000000000000 ) ;
#6906=VERTEX_POINT ( 'NONE', #12865 ) ;
#6909=DIRECTION ( 'NONE',  ( 1.387778780781446169E-16, -1.000000000000000000, -3.469446951953615421E-17 ) ) ;
#6916=CARTESIAN_POINT ( 'NONE',  ( -452.6627218934914367, 399.9999999999998863, -111.4497041420118251 ) ) ;
#6924=DIRECTION ( 'NONE',  ( 0.000000000000000000, 1.000000000000000000, -1.479221584281239571E-31 ) ) ;
#6930=ORIENTED_EDGE ( 'NONE', *, *, #17658, .F. ) ;
#6937=VERTEX_POINT ( 'NONE', #8966 ) ;
#6955=AXIS2_PLACEMENT_3D ( 'NONE', #53845, #5663, #38379 ) ;
#6971=ADVANCED_FACE ( 'NONE', ( #9304 ), #40616, .F. ) ;
#6999=VECTOR ( 'NONE', #38253, 1000.000000000000000 ) ;
#7046=DIRECTION ( 'NONE',  ( 0.000000000000000000, -6.779273404243065824E-32, 1.000000000000000000 ) ) ;
#7117=EDGE_CURVE ( 'NONE', #62102, #66740, #10329, .T. ) ;
#7134=ORIENTED_EDGE ( 'NONE', *, *, #30790, .T. ) ;
#7159=CARTESIAN_POINT ( 'NONE',  ( 417.3372781065083359, 395.0000000000041496, 83.55029585798409641 ) ) ;
#7176=EDGE_LOOP ( 'NONE', ( #35574, #21592, #8229, #16800 ) ) ;
#7180=CYLINDRICAL_SURFACE ( 'NONE', #3091, 5.000000000000004441 ) ;
#7183=CARTESIAN_POINT ( 'NONE',  ( -447.6627218934913799, 0.000000000000000000, -136.4497041420118251 ) ) ;
#7222=CARTESIAN_POINT ( 'NONE',  ( 424.8372781065087906, 400.0000000000044906, 91.05029585798442326 ) ) ;
#7228=CARTESIAN_POINT ( 'NONE',  ( -442.6627218934913799, 0.000000000000000000, -141.4497041420118251 ) ) ;
#7279=LINE ( 'NONE', #23466, #21652 ) ;
#7293=DIRECTION ( 'NONE',  ( 1.000000000000000000, -9.109522253334613014E-16, 0.000000000000000000 ) ) ;
#7312=AXIS2_PLACEMENT_3D ( 'NONE', #27017, #26344, #5225 ) ;
#7337=EDGE_CURVE ( 'NONE', #4215, #59386, #23596, .T. ) ;
#7338=SURFACE_STYLE_USAGE ( .BOTH. , #29476 ) ;
#7355=DIRECTION ( 'NONE',  ( -1.387778780781445922E-16, 1.000000000000000000, 1.232595164407830946E-32 ) ) ;
#7359=VECTOR ( 'NONE', #17917, 1000.000000000000000 ) ;
#7362=VERTEX_POINT ( 'NONE', #48899 ) ;
#7375=AXIS2_PLACEMENT_3D ( 'NONE', #31806, #5064, #26872 ) ;
#7378=EDGE_LOOP ( 'NONE', ( #21724, #53130, #68863, #58672, #15806, #61886, #10687, #5005, #35671, #19994 ) ) ;
#7387=VERTEX_POINT ( 'NONE', #60169 ) ;
#7398=VECTOR ( 'NONE', #8286, 1000.000000000000000 ) ;
#7413=CARTESIAN_POINT ( 'NONE',  ( -447.6627218934918915, 390.0000000000064801, -141.4497041420121377 ) ) ;
#7449=ORIENTED_EDGE ( 'NONE', *, *, #35496, .T. ) ;
#7498=PLANE ( 'NONE',  #46322 ) ;
#7513=ORIENTED_EDGE ( 'NONE', *, *, #35651, .T. ) ;
#7525=VECTOR ( 'NONE', #52717, 1000.000000000000000 ) ;
#7530=CARTESIAN_POINT ( 'NONE',  ( -452.6627218934913230, 217.8591479523843475, 78.55029585798814651 ) ) ;
#7569=VERTEX_POINT ( 'NONE', #65640 ) ;
#7573=AXIS2_PLACEMENT_3D ( 'NONE', #64586, #28334, #69502 ) ;
#7590=DIRECTION ( 'NONE',  ( -1.020422603260505347E-14, 1.000000000000000000, 5.551115123125782702E-17 ) ) ;
#7610=DIRECTION ( 'NONE',  ( 1.850371928290090422E-16, -1.000000000000000000, -1.110223024625156171E-16 ) ) ;
#7612=CARTESIAN_POINT ( 'NONE',  ( -452.6627218934913230, 1.665334536937734811E-13, 78.55029585798817493 ) ) ;
#7613=EDGE_CURVE ( 'NONE', #12229, #61561, #8473, .T. ) ;
#7618=DIRECTION ( 'NONE',  ( -1.000000000000000000, -1.232595164407830946E-32, 1.387778780781445676E-15 ) ) ;
#7621=ORIENTED_EDGE ( 'NONE', *, *, #46703, .F. ) ;
#7635=CARTESIAN_POINT ( 'NONE',  ( -452.6627218934913230, 1.665334536937734811E-13, 113.5502958579881749 ) ) ;
#7644=EDGE_CURVE ( 'NONE', #16629, #65265, #45914, .T. ) ;
#7645=CARTESIAN_POINT ( 'NONE',  ( 112.3013380801408658, 400.0000000000066507, -128.9497041420121093 ) ) ;
#7695=DIRECTION ( 'NONE',  ( -1.604841615724188478E-15, -1.000000000000000000, -1.236108373964834415E-14 ) ) ;
#7707=CARTESIAN_POINT ( 'NONE',  ( -452.6627218934859229, 390.0000000000064801, -136.4497041420121661 ) ) ;
#7741=ADVANCED_FACE ( 'NONE', ( #10341 ), #11032, .T. ) ;
#7797=LINE ( 'NONE', #50700, #3590 ) ;
#7804=CIRCLE ( 'NONE', #25785, 5.000000000000004441 ) ;
#7808=PLANE ( 'NONE',  #52124 ) ;
#7817=VECTOR ( 'NONE', #28, 1000.000000000000000 ) ;
#7822=DIRECTION ( 'NONE',  ( -1.000000000000000000, -1.387778780781448141E-16, 5.551115123125781716E-16 ) ) ;
#7825=( BOUNDED_CURVE ( )  B_SPLINE_CURVE ( 3, ( #27691, #33341, #17487, #29102 ),
 .UNSPECIFIED., .F., .F. ) 
 B_SPLINE_CURVE_WITH_KNOTS ( ( 4, 4 ),
 ( 1.570796326794896558, 3.141592653589793116 ),
 .UNSPECIFIED. ) 
 CURVE ( )  GEOMETRIC_REPRESENTATION_ITEM ( )  RATIONAL_B_SPLINE_CURVE ( ( 1.000000000000000000, 0.8047378541243649375, 0.8047378541243649375, 1.000000000000000000 ) ) 
 REPRESENTATION_ITEM ( '' )  );
#7826=FACE_OUTER_BOUND ( 'NONE', #51753, .T. ) ;
#7846=ORIENTED_EDGE ( 'NONE', *, *, #15818, .T. ) ;
#7866=DIRECTION ( 'NONE',  ( 1.000000000000000000, 0.000000000000000000, 2.775557561562796688E-15 ) ) ;
#7875=VERTEX_POINT ( 'NONE', #23687 ) ;
#7883=DIRECTION ( 'NONE',  ( 0.000000000000000000, -7.395570986446983486E-32, -1.000000000000000000 ) ) ;
#7884=VECTOR ( 'NONE', #4400, 1000.000000000000000 ) ;
#7893=FACE_OUTER_BOUND ( 'NONE', #22120, .T. ) ;
#7978=VECTOR ( 'NONE', #16221, 1000.000000000000000 ) ;
#7980=CARTESIAN_POINT ( 'NONE',  ( -452.6627218934913230, 399.9999999999997726, 83.55029585798818914 ) ) ;
#7983=ORIENTED_EDGE ( 'NONE', *, *, #21537, .T. ) ;
#8003=VERTEX_POINT ( 'NONE', #30347 ) ;
#8023=SURFACE_STYLE_FILL_AREA ( #55511 ) ;
#8038=( LENGTH_UNIT ( ) NAMED_UNIT ( * ) SI_UNIT ( .MILLI., .METRE. ) );
#8064=PRODUCT ( 'frame_Default<As Welded>', 'frame_Default<As Welded>', '', ( #42401 ) ) ;
#8068=AXIS2_PLACEMENT_3D ( 'NONE', #25370, #68274, #68936 ) ;
#8075=LINE ( 'NONE', #9466, #16183 ) ;
#8076=CLOSED_SHELL ( 'NONE', ( #37480, #10315, #4132, #35670, #17211, #17781, #51490, #4050, #57996, #4458, #3784, #15788, #54123, #26352, #31839, #51393, #39881, #55191, #16444 ) ) ;
#8078=EDGE_CURVE ( 'NONE', #41137, #60705, #62355, .T. ) ;
#8095=DIRECTION ( 'NONE',  ( -3.081487911019579554E-32, -1.000000000000000000, -3.469446951953612956E-17 ) ) ;
#8112=PLANE ( 'NONE',  #2250 ) ;
#8130=EDGE_CURVE ( 'NONE', #18081, #10959, #45047, .T. ) ;
#8135=EDGE_LOOP ( 'NONE', ( #60055, #64218, #25337, #33874 ) ) ;
#8140=FACE_OUTER_BOUND ( 'NONE', #18034, .T. ) ;
#8160=ORIENTED_EDGE ( 'NONE', *, *, #47994, .F. ) ;
#8171=VERTEX_POINT ( 'NONE', #23949 ) ;
#8229=ORIENTED_EDGE ( 'NONE', *, *, #37636, .F. ) ;
#8249=DIRECTION ( 'NONE',  ( 1.000000000000000000, 1.001918046209079887E-14, -9.729495617646301779E-15 ) ) ;
#8286=DIRECTION ( 'NONE',  ( -1.000000000000000000, 9.109522253334613014E-16, 1.697894969632810648E-16 ) ) ;
#8305=LINE ( 'NONE', #20836, #15087 ) ;
#8319=DIRECTION ( 'NONE',  ( 1.000000000000000000, 0.000000000000000000, 0.000000000000000000 ) ) ;
#8356=ORIENTED_EDGE ( 'NONE', *, *, #68983, .T. ) ;
#8396=CARTESIAN_POINT ( 'NONE',  ( -447.6627218934913799, 367.0710678118653050, -141.4497041420117966 ) ) ;
#8401=ORIENTED_EDGE ( 'NONE', *, *, #21582, .F. ) ;
#8405=ORIENTED_EDGE ( 'NONE', *, *, #38999, .T. ) ;
#8418=AXIS2_PLACEMENT_3D ( 'NONE', #21280, #53272, #5101 ) ;
#8426=DIRECTION ( 'NONE',  ( -4.270088556250601699E-16, -0.000000000000000000, -1.000000000000000000 ) ) ;
#8435=AXIS2_PLACEMENT_3D ( 'NONE', #12625, #55524, #7355 ) ;
#8473=CIRCLE ( 'NONE', #47765, 5.000000000000060396 ) ;
#8526=EDGE_CURVE ( 'NONE', #38085, #19443, #14002, .T. ) ;
#8527=VERTEX_POINT ( 'NONE', #29143 ) ;
#8538=CARTESIAN_POINT ( 'NONE',  ( -444.2277112916228248, 394.7494927581580555, -127.5188852347322666 ) ) ;
#8546=DIRECTION ( 'NONE',  ( 1.000000000000000000, 1.850550996349095901E-16, 1.228197773518735191E-20 ) ) ;
#8556=DIRECTION ( 'NONE',  ( 1.000000000000000000, 1.387778780781443950E-16, 0.000000000000000000 ) ) ;
#8557=ORIENTED_EDGE ( 'NONE', *, *, #41327, .T. ) ;
#8581=UNCERTAINTY_MEASURE_WITH_UNIT (LENGTH_MEASURE( 1.000000000000000082E-05 ), #28794, 'distance_accuracy_value', 'NONE');
#8630=CYLINDRICAL_SURFACE ( 'NONE', #46665, 5.000000000000087930 ) ;
#8662=AXIS2_PLACEMENT_3D ( 'NONE', #64980, #28378, #22756 ) ;
#8670=VECTOR ( 'NONE', #66113, 1000.000000000000000 ) ;
#8681=EDGE_CURVE ( 'NONE', #7362, #46731, #15214, .T. ) ;
#8703=VECTOR ( 'NONE', #34561, 1000.000000000000000 ) ;
#8717=ORIENTED_EDGE ( 'NONE', *, *, #39789, .F. ) ;
#8729=LINE ( 'NONE', #9412, #65502 ) ;
#8732=DIRECTION ( 'NONE',  ( -4.314083075427411048E-32, -1.000000000000000000, -6.123233995736763571E-17 ) ) ;
#8787=DIRECTION ( 'NONE',  ( -0.7071067811865405783, -7.105427357601001070E-15, 0.7071067811865545671 ) ) ;
#8838=EDGE_LOOP ( 'NONE', ( #21577, #35325, #6890, #57481 ) ) ;
#8849=DIRECTION ( 'NONE',  ( 1.000000000000000000, 0.000000000000000000, 0.000000000000000000 ) ) ;
#8856=DIRECTION ( 'NONE',  ( -1.000000000000000000, -1.387778780781446415E-16, 0.000000000000000000 ) ) ;
#8887=DIRECTION ( 'NONE',  ( -1.850169831522831466E-16, 1.000000000000000000, 1.110223024625156294E-16 ) ) ;
#8890=DIRECTION ( 'NONE',  ( -1.110223024625156047E-16, -1.000000000000000000, -1.110223024625155678E-16 ) ) ;
#8899=CARTESIAN_POINT ( 'NONE',  ( 437.3372781065086201, 0.000000000000000000, 103.5502958579881749 ) ) ;
#8916=ORIENTED_EDGE ( 'NONE', *, *, #6659, .T. ) ;
#8966=CARTESIAN_POINT ( 'NONE',  ( 50.98853755884157124, 395.0000000000065938, -133.9497041420122798 ) ) ;
#8970=CARTESIAN_POINT ( 'NONE',  ( 417.3372781065085633, 395.0000000000000568, -146.4497041420118535 ) ) ;
#8973=VERTEX_POINT ( 'NONE', #9512 ) ;
#8986=ORIENTED_EDGE ( 'NONE', *, *, #28519, .F. ) ;
#8992=AXIS2_PLACEMENT_3D ( 'NONE', #40810, #34519, #67555 ) ;
#9011=ADVANCED_FACE ( 'NONE', ( #37261 ), #26724, .F. ) ;
#9014=VERTEX_POINT ( 'NONE', #36937 ) ;
#9018=CARTESIAN_POINT ( 'NONE',  ( 429.8372781065087906, 395.0000000000066507, -128.9497041420121093 ) ) ;
#9046=ORIENTED_EDGE ( 'NONE', *, *, #49061, .F. ) ;
#9091=ORIENTED_EDGE ( 'NONE', *, *, #1996, .T. ) ;
#9093=ORIENTED_EDGE ( 'NONE', *, *, #15435, .F. ) ;
#9108=VERTEX_POINT ( 'NONE', #64008 ) ;
#9136=ORIENTED_EDGE ( 'NONE', *, *, #1352, .F. ) ;
#9149=VERTEX_POINT ( 'NONE', #44978 ) ;
#9156=CARTESIAN_POINT ( 'NONE',  ( -442.6627218934913230, 399.9999999999997726, 103.5502958579881891 ) ) ;
#9168=VECTOR ( 'NONE', #59971, 1000.000000000000000 ) ;
#9188=VERTEX_POINT ( 'NONE', #17189 ) ;
#9195=DIRECTION ( 'NONE',  ( 1.000000000000000000, 1.110223024625118675E-14, -1.110223024625118675E-14 ) ) ;
#9220=CARTESIAN_POINT ( 'NONE',  ( -444.4229916354184979, 394.6798985497181889, -128.5895624939293498 ) ) ;
#9231=DIRECTION ( 'NONE',  ( 1.000000000000000000, 1.387778780781445676E-16, 0.000000000000000000 ) ) ;
#9246=CARTESIAN_POINT ( 'NONE',  ( -449.7337897053571965, 364.9999999999955662, 110.6213636698579705 ) ) ;
#9251=DIRECTION ( 'NONE',  ( 0.7071067811865405783, 7.105427357601001070E-15, -0.7071067811865545671 ) ) ;
#9258=UNCERTAINTY_MEASURE_WITH_UNIT (LENGTH_MEASURE( 1.000000000000000082E-05 ), #38027, 'distance_accuracy_value', 'NONE');
#9261=CARTESIAN_POINT ( 'NONE',  ( -417.6627218934913230, 219.4906275429376308, -144.4497041420118819 ) ) ;
#9271=ORIENTED_EDGE ( 'NONE', *, *, #49208, .T. ) ;
#9304=FACE_OUTER_BOUND ( 'NONE', #4348, .T. ) ;
#9315=DIRECTION ( 'NONE',  ( 0.7071067811865476838, -6.441404958702661839E-16, 0.7071067811865474617 ) ) ;
#9318=DIRECTION ( 'NONE',  ( 0.000000000000000000, -0.000000000000000000, 1.000000000000000000 ) ) ;
#9339=DIRECTION ( 'NONE',  ( 0.7071067811865473507, -6.441404958702665783E-16, -0.7071067811865477948 ) ) ;
#9372=ORIENTED_EDGE ( 'NONE', *, *, #27484, .T. ) ;
#9399=EDGE_CURVE ( 'NONE', #17356, #57474, #31288, .T. ) ;
#9409=COLOUR_RGB ( '',0.7921568627450980005, 0.8196078431372548767, 0.9333333333333333481 ) ;
#9412=CARTESIAN_POINT ( 'NONE',  ( 442.3372781065085633, 400.0000000000000568, -136.4497041420118251 ) ) ;
#9413=VECTOR ( 'NONE', #11666, 1000.000000000000000 ) ;
#9430=DIRECTION ( 'NONE',  ( -0.000000000000000000, 0.000000000000000000, -1.000000000000000000 ) ) ;
#9432=CARTESIAN_POINT ( 'NONE',  ( 50.98853755884142203, 395.0000000000065938, -123.9497041420120382 ) ) ;
#9454=EDGE_CURVE ( 'NONE', #32748, #26944, #30593, .T. ) ;
#9466=CARTESIAN_POINT ( 'NONE',  ( -440.1146514826279486, 388.0000000000019895, 101.0022254471289074 ) ) ;
#9504=VECTOR ( 'NONE', #6347, 1000.000000000000000 ) ;
#9512=CARTESIAN_POINT ( 'NONE',  ( 442.3372781065086201, 0.000000000000000000, 83.55029585798817493 ) ) ;
#9563=ORIENTED_EDGE ( 'NONE', *, *, #3366, .F. ) ;
#9569=VECTOR ( 'NONE', #16116, 1000.000000000000000 ) ;
#9570=CARTESIAN_POINT ( 'NONE',  ( -443.6229740799757906, 394.9118408295729523, -126.2130497528550990 ) ) ;
#9621=CARTESIAN_POINT ( 'NONE',  ( 424.8372781065089043, 400.0000000000000568, -123.9497041420121235 ) ) ;
#9626=EDGE_LOOP ( 'NONE', ( #30057, #38468, #49736, #30287 ) ) ;
#9643=ORIENTED_EDGE ( 'NONE', *, *, #37934, .F. ) ;
#9659=ORIENTED_EDGE ( 'NONE', *, *, #26286, .F. ) ;
#9666=DIRECTION ( 'NONE',  ( 1.000000000000000000, 1.131929979755206441E-16, -1.697894969632809662E-16 ) ) ;
#9670=( BOUNDED_CURVE ( )  B_SPLINE_CURVE ( 3, ( #66116, #44977, #39359, #66459 ),
 .UNSPECIFIED., .F., .F. ) 
 B_SPLINE_CURVE_WITH_KNOTS ( ( 4, 4 ),
 ( 1.570796326794908326, 3.141592653589805106 ),
 .UNSPECIFIED. ) 
 CURVE ( )  GEOMETRIC_REPRESENTATION_ITEM ( )  RATIONAL_B_SPLINE_CURVE ( ( 1.000000000000000000, 0.8047378541243649375, 0.8047378541243649375, 1.000000000000000000 ) ) 
 REPRESENTATION_ITEM ( '' )  );
#9717=AXIS2_PLACEMENT_3D ( 'NONE', #36878, #25295, #57642 ) ;
#9718=AXIS2_PLACEMENT_3D ( 'NONE', #5384, #63791, #26840 ) ;
#9734=PLANE ( 'NONE',  #26091 ) ;
#9766=ORIENTED_EDGE ( 'NONE', *, *, #67198, .F. ) ;
#9770=CARTESIAN_POINT ( 'NONE',  ( 433.3728120124414431, 400.0000000000110276, 99.58582976391696207 ) ) ;
#9775=PLANE ( 'NONE',  #21503 ) ;
#9780=ORIENTED_EDGE ( 'NONE', *, *, #63242, .F. ) ;
#9832=ADVANCED_FACE ( 'NONE', ( #10766 ), #11445, .F. ) ;
#9847=EDGE_CURVE ( 'NONE', #54476, #45879, #32233, .T. ) ;
#9854=LINE ( 'NONE', #31311, #54269 ) ;
#9866=CARTESIAN_POINT ( 'NONE',  ( -440.1146514826279486, 388.0000000000064233, 101.0022254471246441 ) ) ;
#9868=ORIENTED_EDGE ( 'NONE', *, *, #57601, .T. ) ;
#9889=CARTESIAN_POINT ( 'NONE',  ( 412.3372781065086770, 0.000000000000000000, -146.4497041420118251 ) ) ;
#9936=CARTESIAN_POINT ( 'NONE',  ( -442.6627218934912662, 394.9999999999998295, 92.24186470396634263 ) ) ;
#9937=VERTEX_POINT ( 'NONE', #28698 ) ;
#9942=CARTESIAN_POINT ( 'NONE',  ( -305.1627218934913230, 399.9999999999997726, 1.050295857988214898 ) ) ;
#9956=CARTESIAN_POINT ( 'NONE',  ( 417.3372781065086201, 399.9999999999998863, 108.5502958579881891 ) ) ;
#9994=ORIENTED_EDGE ( 'NONE', *, *, #48174, .F. ) ;
#10003=DIRECTION ( 'NONE',  ( 1.000000000000000000, 0.000000000000000000, 1.337618101958020291E-16 ) ) ;
#10008=LINE ( 'NONE', #20903, #62599 ) ;
#10011=LINE ( 'NONE', #53586, #17031 ) ;
#10089=EDGE_CURVE ( 'NONE', #61561, #24336, #57847, .T. ) ;
#10094=CARTESIAN_POINT ( 'NONE',  ( 50.98853755884132255, 395.0000000000004547, 91.05029585798797598 ) ) ;
#10119=( NAMED_UNIT ( * ) SI_UNIT ( $, .STERADIAN. ) SOLID_ANGLE_UNIT ( ) );
#10134=EDGE_CURVE ( 'NONE', #26715, #7387, #10008, .T. ) ;
#10145=ORIENTED_EDGE ( 'NONE', *, *, #28172, .F. ) ;
#10155=EDGE_CURVE ( 'NONE', #36914, #55296, #19875, .T. ) ;
#10194=CARTESIAN_POINT ( 'NONE',  ( 424.8372781065089612, 400.0000000000001705, 91.05029585798857283 ) ) ;
#10207=DIRECTION ( 'NONE',  ( 1.000000000000000000, 1.110223024625118675E-14, -1.110223024625118675E-14 ) ) ;
#10210=ADVANCED_FACE ( 'NONE', ( #58866 ), #54267, .T. ) ;
#10223=EDGE_CURVE ( 'NONE', #38457, #366, #26527, .T. ) ;
#10233=ADVANCED_FACE ( 'NONE', ( #44071 ), #59899, .F. ) ;
#10239=CARTESIAN_POINT ( 'NONE',  ( 412.3372781065085064, 397.0710678118653618, 78.55029585798826020 ) ) ;
#10254=CARTESIAN_POINT ( 'NONE',  ( 447.3372781065082791, 400.0000000000044338, 78.55029585798382641 ) ) ;
#10262=ORIENTED_EDGE ( 'NONE', *, *, #44657, .F. ) ;
#10270=AXIS2_PLACEMENT_3D ( 'NONE', #36324, #20830, #58124 ) ;
#10278=CARTESIAN_POINT ( 'NONE',  ( -422.6627218934914367, 0.000000000000000000, -141.4497041420118535 ) ) ;
#10294=CYLINDRICAL_SURFACE ( 'NONE', #60867, 5.000000000000060396 ) ;
#10304=EDGE_CURVE ( 'NONE', #56564, #55579, #27908, .T. ) ;
#10315=ADVANCED_FACE ( 'NONE', ( #39512 ), #17714, .F. ) ;
#10318=CLOSED_SHELL ( 'NONE', ( #44388, #64080, #1409, #13631, #52648, #31992 ) ) ;
#10322=CARTESIAN_POINT ( 'NONE',  ( 50.98853755884157124, 400.0000000000065938, -128.9497041420121946 ) ) ;
#10326=LINE ( 'NONE', #20890, #66259 ) ;
#10329=LINE ( 'NONE', #53577, #15241 ) ;
#10338=CARTESIAN_POINT ( 'NONE',  ( 107.3013380801406385, 400.0000000000076739, 96.05029585798752123 ) ) ;
#10341=FACE_OUTER_BOUND ( 'NONE', #30220, .T. ) ;
#10347=DIRECTION ( 'NONE',  ( -1.000000000000000000, -0.000000000000000000, -0.000000000000000000 ) ) ;
#10356=ORIENTED_EDGE ( 'NONE', *, *, #817, .F. ) ;
#10364=DIRECTION ( 'NONE',  ( 1.000000000000000000, 1.110223024625155594E-14, -1.110223024625155594E-14 ) ) ;
#10370=FACE_OUTER_BOUND ( 'NONE', #17033, .T. ) ;
#10373=DIRECTION ( 'NONE',  ( -3.081487911019579554E-32, -1.000000000000000000, -3.469446951953612956E-17 ) ) ;
#10466=EDGE_CURVE ( 'NONE', #61415, #55296, #4632, .T. ) ;
#10470=CARTESIAN_POINT ( 'NONE',  ( 442.3372781065085633, 392.9289321881346382, -141.4497041420117966 ) ) ;
#10482=CARTESIAN_POINT ( 'NONE',  ( 112.3013380801408658, 400.0000000000065938, 91.05029585798857283 ) ) ;
#10505=AXIS2_PLACEMENT_3D ( 'NONE', #28042, #11863, #7293 ) ;
#10531=DIRECTION ( 'NONE',  ( 1.334402673828311860E-15, -1.000000000000000000, 0.000000000000000000 ) ) ;
#10536=ADVANCED_FACE ( 'NONE', ( #68988 ), #13807, .T. ) ;
#10538=LINE ( 'NONE', #10194, #67172 ) ;
#10548=CYLINDRICAL_SURFACE ( 'NONE', #59281, 5.000000000000004441 ) ;
#10550=VECTOR ( 'NONE', #46109, 1000.000000000000000 ) ;
#10558=EDGE_CURVE ( 'NONE', #4675, #15602, #15496, .T. ) ;
#10563=AXIS2_PLACEMENT_3D ( 'NONE', #2956, #45504, #66989 ) ;
#10597=CARTESIAN_POINT ( 'NONE',  ( 447.3372781065085633, 365.0000000000001137, -146.4497041420118251 ) ) ;
#10610=PRESENTATION_STYLE_ASSIGNMENT (( #4649 ) ) ;
#10619=EDGE_LOOP ( 'NONE', ( #31894, #45676, #45909, #49439 ) ) ;
#10648=ORIENTED_EDGE ( 'NONE', *, *, #61789, .T. ) ;
#10687=ORIENTED_EDGE ( 'NONE', *, *, #11964, .T. ) ;
#10723=EDGE_LOOP ( 'NONE', ( #13621, #18710, #52372, #18212 ) ) ;
#10745=AXIS2_PLACEMENT_3D ( 'NONE', #21102, #62970, #52070 ) ;
#10753=VECTOR ( 'NONE', #44699, 1000.000000000000000 ) ;
#10766=FACE_OUTER_BOUND ( 'NONE', #35088, .T. ) ;
#10781=CARTESIAN_POINT ( 'NONE',  ( 429.8372781065087338, 388.0000000000066507, -123.9497041420121235 ) ) ;
#10801=VERTEX_POINT ( 'NONE', #14676 ) ;
#10836=ORIENTED_EDGE ( 'NONE', *, *, #49373, .T. ) ;
#10845=LINE ( 'NONE', #4203, #21559 ) ;
#10847=AXIS2_PLACEMENT_3D ( 'NONE', #32459, #53550, #32117 ) ;
#10876=CARTESIAN_POINT ( 'NONE',  ( 412.3372781065085633, 400.0000000000000568, -111.4497041420117682 ) ) ;
#10886=ORIENTED_EDGE ( 'NONE', *, *, #65532, .F. ) ;
#10908=DIRECTION ( 'NONE',  ( 1.000000000000000000, 1.387778780781445922E-16, 0.000000000000000000 ) ) ;
#10926=CARTESIAN_POINT ( 'NONE',  ( -444.4229916354184979, 394.6798985497181320, 96.05029585798874336 ) ) ;
#10959=VERTEX_POINT ( 'NONE', #33646 ) ;
#10995=FACE_OUTER_BOUND ( 'NONE', #10723, .T. ) ;
#11032=PLANE ( 'NONE',  #7375 ) ;
#11048=LINE ( 'NONE', #32509, #50557 ) ;
#11052=ORIENTED_EDGE ( 'NONE', *, *, #53882, .F. ) ;
#11063=CARTESIAN_POINT ( 'NONE',  ( -422.6627218934914367, 0.000000000000000000, -146.4497041420118251 ) ) ;
#11064=CARTESIAN_POINT ( 'NONE',  ( -444.4229916354184979, 394.6798985497180752, -129.3091912309550935 ) ) ;
#11070=SHAPE_DEFINITION_REPRESENTATION ( #55795, #2894 ) ;
#11083=ORIENTED_EDGE ( 'NONE', *, *, #45213, .F. ) ;
#11114=CARTESIAN_POINT ( 'NONE',  ( -430.1627218934916073, 399.9999999999998863, -123.9497041420119530 ) ) ;
#11116=LINE ( 'NONE', #37856, #66202 ) ;
#11117=LINE ( 'NONE', #26271, #68809 ) ;
#11146=CYLINDRICAL_SURFACE ( 'NONE', #64538, 5.000000000000004441 ) ;
#11214=DIRECTION ( 'NONE',  ( 0.7071067811865474617, 9.058225723175622340E-16, -0.7071067811865474617 ) ) ;
#11229=CARTESIAN_POINT ( 'NONE',  ( 442.3372781065085633, 395.0000000000001137, -141.4497041420118251 ) ) ;
#11260=EDGE_LOOP ( 'NONE', ( #56105, #28464, #10356, #52863 ) ) ;
#11264=DIRECTION ( 'NONE',  ( 1.387778780781445922E-16, -1.000000000000000000, -1.232595164407830946E-32 ) ) ;
#11270=CARTESIAN_POINT ( 'NONE',  ( -442.9409111889697215, 394.9999999999998863, 99.62207883810852138 ) ) ;
#11273=LINE ( 'NONE', #31369, #39250 ) ;
#11275=CARTESIAN_POINT ( 'NONE',  ( -439.4229916354183274, 388.0000000000064233, 96.05029585798874336 ) ) ;
#11292=EDGE_LOOP ( 'NONE', ( #36058, #8717, #26015, #4098 ) ) ;
#11341=ORIENTED_EDGE ( 'NONE', *, *, #28573, .T. ) ;
#11343=DIRECTION ( 'NONE',  ( -1.000000000000000000, -1.001918829714556097E-14, 9.899279560275163638E-15 ) ) ;
#11346=EDGE_LOOP ( 'NONE', ( #40918, #19517, #66865, #43879 ) ) ;
#11349=AXIS2_PLACEMENT_3D ( 'NONE', #23558, #44995, #66478 ) ;
#11369=DIRECTION ( 'NONE',  ( 0.000000000000000000, -1.000000000000000000, -1.110223024625156171E-16 ) ) ;
#11406=AXIS2_PLACEMENT_3D ( 'NONE', #9156, #42198, #15469 ) ;
#11445=CYLINDRICAL_SURFACE ( 'NONE', #7573, 5.000000000000004441 ) ;
#11482=ORIENTED_EDGE ( 'NONE', *, *, #49312, .F. ) ;
#11485=ADVANCED_FACE ( 'NONE', ( #15562 ), #4650, .T. ) ;
#11489=EDGE_CURVE ( 'NONE', #36015, #6906, #35979, .T. ) ;
#11499=CARTESIAN_POINT ( 'NONE',  ( 437.3372781065086201, 0.000000000000000000, -141.4497041420118251 ) ) ;
#11526=CARTESIAN_POINT ( 'NONE',  ( 412.3372781065085633, 219.4906275429376308, -146.4497041420117682 ) ) ;
#11540=EDGE_CURVE ( 'NONE', #68125, #66740, #31266, .T. ) ;
#11554=LINE ( 'NONE', #43215, #35467 ) ;
#11562=LINE ( 'NONE', #33039, #44295 ) ;
#11565=CARTESIAN_POINT ( 'NONE',  ( -447.6627218934918915, 390.0000000000064801, -141.4497041420121377 ) ) ;
#11572=DIRECTION ( 'NONE',  ( 0.7071067811865474617, 9.058225723175622340E-16, -0.7071067811865474617 ) ) ;
#11585=DIRECTION ( 'NONE',  ( 1.020422603260505347E-14, -1.000000000000000000, -5.551115123125782702E-17 ) ) ;
#11609=CIRCLE ( 'NONE', #65516, 5.000000000000060396 ) ;
#11625=ORIENTED_EDGE ( 'NONE', *, *, #6427, .F. ) ;
#11626=DIRECTION ( 'NONE',  ( -9.109522253334603153E-16, -1.000000000000000000, -9.109522253334599209E-16 ) ) ;
#11648=MECHANICAL_DESIGN_GEOMETRIC_PRESENTATION_REPRESENTATION('',(#63384),#45406);
#11658=VECTOR ( 'NONE', #32677, 1000.000000000000000 ) ;
#11666=DIRECTION ( 'NONE',  ( 1.000000000000000000, 1.387778780781446908E-16, 0.000000000000000000 ) ) ;
#11670=CARTESIAN_POINT ( 'NONE',  ( -450.6627218934913230, 177.8591479523843475, 78.55029585798814651 ) ) ;
#11671=ORIENTED_EDGE ( 'NONE', *, *, #66153, .T. ) ;
#11675=DIRECTION ( 'NONE',  ( 0.000000000000000000, 4.930380657631322689E-32, 1.000000000000000000 ) ) ;
#11688=EDGE_LOOP ( 'NONE', ( #68596, #34512, #59088, #39837 ) ) ;
#11706=DIRECTION ( 'NONE',  ( 0.7071067811865473507, -6.441404958702665783E-16, -0.7071067811865477948 ) ) ;
#11742=VERTEX_POINT ( 'NONE', #18329 ) ;
#11744=CARTESIAN_POINT ( 'NONE',  ( -452.6627218934914367, 399.9999999999998863, -146.4497041420118251 ) ) ;
#11753=AXIS2_PLACEMENT_3D ( 'NONE', #26484, #5702, #31417 ) ;
#11758=DIRECTION ( 'NONE',  ( -1.850169831522831466E-16, 1.000000000000000000, 1.110223024625156294E-16 ) ) ;
#11759=PLANE ( 'NONE',  #8418 ) ;
#11791=VECTOR ( 'NONE', #17720, 1000.000000000000000 ) ;
#11794=LINE ( 'NONE', #42430, #6187 ) ;
#11801=AXIS2_PLACEMENT_3D ( 'NONE', #52268, #41025, #62482 ) ;
#11804=DIRECTION ( 'NONE',  ( -1.850169831522831466E-16, 1.000000000000000000, 1.110223024625156294E-16 ) ) ;
#11844=ORIENTED_EDGE ( 'NONE', *, *, #7613, .T. ) ;
#11856=LINE ( 'NONE', #34023, #28999 ) ;
#11863=DIRECTION ( 'NONE',  ( -9.109522253334613014E-16, -1.000000000000000000, 3.889846672687432470E-31 ) ) ;
#11896=VERTEX_POINT ( 'NONE', #3207 ) ;
#11920=CARTESIAN_POINT ( 'NONE',  ( 442.3372781065085633, 395.0000000000001137, -141.4497041420118251 ) ) ;
#11940=VERTEX_POINT ( 'NONE', #30281 ) ;
#11945=CARTESIAN_POINT ( 'NONE',  ( -417.6627218934913799, 0.000000000000000000, -146.4497041420118251 ) ) ;
#11957=CARTESIAN_POINT ( 'NONE',  ( 412.3372781065085633, 179.4906275429376024, -144.4497041420117682 ) ) ;
#11964=EDGE_CURVE ( 'NONE', #36942, #9188, #46862, .T. ) ;
#11973=ORIENTED_EDGE ( 'NONE', *, *, #38417, .F. ) ;
#11986=DIRECTION ( 'NONE',  ( -1.000000000000000000, 0.000000000000000000, 0.000000000000000000 ) ) ;
#12005=ORIENTED_EDGE ( 'NONE', *, *, #21449, .T. ) ;
#12014=ADVANCED_FACE ( 'NONE', ( #47818 ), #37257, .T. ) ;
#12021=ORIENTED_EDGE ( 'NONE', *, *, #47787, .F. ) ;
#12052=VECTOR ( 'NONE', #17020, 1000.000000000000000 ) ;
#12077=EDGE_CURVE ( 'NONE', #52163, #34907, #60800, .T. ) ;
#12094=VERTEX_POINT ( 'NONE', #40053 ) ;
#12162=EDGE_CURVE ( 'NONE', #59386, #13106, #39256, .T. ) ;
#12164=LINE ( 'NONE', #39588, #30963 ) ;
#12174=AXIS2_PLACEMENT_3D ( 'NONE', #16240, #54557, #17276 ) ;
#12184=LINE ( 'NONE', #39608, #26178 ) ;
#12208=CYLINDRICAL_SURFACE ( 'NONE', #56816, 5.000000000000170530 ) ;
#12220=VERTEX_POINT ( 'NONE', #46353 ) ;
#12229=VERTEX_POINT ( 'NONE', #30199 ) ;
#12240=EDGE_LOOP ( 'NONE', ( #41352, #43715, #51214, #45345 ) ) ;
#12243=LINE ( 'NONE', #23146, #31562 ) ;
#12247=DIRECTION ( 'NONE',  ( 0.000000000000000000, -1.000000000000000000, 0.000000000000000000 ) ) ;
#12257=VECTOR ( 'NONE', #61557, 1000.000000000000000 ) ;
#12272=ORIENTED_EDGE ( 'NONE', *, *, #38557, .T. ) ;
#12285=DIRECTION ( 'NONE',  ( -1.850169831522831466E-16, 1.000000000000000000, 1.110223024625156294E-16 ) ) ;
#12299=CARTESIAN_POINT ( 'NONE',  ( 429.8372781065087338, 400.0000000000066507, 91.05029585798857283 ) ) ;
#12303=ADVANCED_FACE ( 'NONE', ( #25954 ), #28273, .F. ) ;
#12313=DIRECTION ( 'NONE',  ( -1.000000000000000000, 0.000000000000000000, 0.000000000000000000 ) ) ;
#12320=ORIENTED_EDGE ( 'NONE', *, *, #50891, .T. ) ;
#12327=CARTESIAN_POINT ( 'NONE',  ( 417.3372781065086770, 0.000000000000000000, 113.5502958579881749 ) ) ;
#12331=( BOUNDED_CURVE ( )  B_SPLINE_CURVE ( 3, ( #16395, #37495, #64233, #62248 ),
 .UNSPECIFIED., .F., .F. ) 
 B_SPLINE_CURVE_WITH_KNOTS ( ( 4, 4 ),
 ( 1.655128935956321114E-13, 1.570796326794890563 ),
 .UNSPECIFIED. ) 
 CURVE ( )  GEOMETRIC_REPRESENTATION_ITEM ( )  RATIONAL_B_SPLINE_CURVE ( ( 1.000000000000000000, 0.8047378541244054606, 0.8047378541244054606, 1.000000000000000000 ) ) 
 REPRESENTATION_ITEM ( '' )  );
#12340=CARTESIAN_POINT ( 'NONE',  ( -417.6627218934914367, 399.9999999999998863, -146.4497041420118251 ) ) ;
#12354=DIRECTION ( 'NONE',  ( 0.000000000000000000, 6.123233995736870806E-17, -1.000000000000000000 ) ) ;
#12369=VERTEX_POINT ( 'NONE', #18086 ) ;
#12388=EDGE_CURVE ( 'NONE', #21328, #1580, #62020, .T. ) ;
#12391=DIRECTION ( 'NONE',  ( 0.7071067811865543451, 7.105427357601001070E-15, 0.7071067811865408004 ) ) ;
#12407=DIRECTION ( 'NONE',  ( 1.000000000000000000, 2.465190328815660250E-32, 0.000000000000000000 ) ) ;
#12408=ADVANCED_FACE ( 'NONE', ( #45852 ), #18426, .T. ) ;
#12414=ADVANCED_FACE ( 'NONE', ( #24410 ), #7180, .F. ) ;
#12432=CYLINDRICAL_SURFACE ( 'NONE', #51812, 5.000000000000004441 ) ;
#12433=CARTESIAN_POINT ( 'NONE',  ( -439.4229916354183274, 388.0000000000064233, 96.05029585798874336 ) ) ;
#12475=DIRECTION ( 'NONE',  ( 1.387778780781446169E-16, -1.000000000000000000, -3.469446951953615421E-17 ) ) ;
#12495=DIRECTION ( 'NONE',  ( 1.000000000000000000, 1.387778780781446908E-16, 0.000000000000000000 ) ) ;
#12499=EDGE_CURVE ( 'NONE', #12094, #56059, #68028, .T. ) ;
#12574=DIRECTION ( 'NONE',  ( -1.000000000000000000, 2.279101714840934323E-64, -7.703719777548945123E-34 ) ) ;
#12578=CARTESIAN_POINT ( 'NONE',  ( 112.3013380801408658, 400.0000000000066507, -133.9497041420121377 ) ) ;
#12582=CARTESIAN_POINT ( 'NONE',  ( -422.6627218934914936, 394.9999999999956799, 83.55029585799226766 ) ) ;
#12584=ADVANCED_FACE ( 'NONE', ( #39069 ), #27446, .F. ) ;
#12625=CARTESIAN_POINT ( 'NONE',  ( -452.6627218934914367, 399.9999999999998863, -111.4497041420118251 ) ) ;
#12637=LINE ( 'NONE', #10278, #44125 ) ;
#12643=VECTOR ( 'NONE', #62882, 1000.000000000000000 ) ;
#12671=VECTOR ( 'NONE', #6342, 1000.000000000000000 ) ;
#12676=VECTOR ( 'NONE', #33989, 1000.000000000000000 ) ;
#12684=AXIS2_PLACEMENT_3D ( 'NONE', #20845, #41961, #42306 ) ;
#12705=EDGE_LOOP ( 'NONE', ( #58243, #17081, #64936, #66962 ) ) ;
#12716=DIRECTION ( 'NONE',  ( 1.697742017499683849E-16, -1.665334536937734564E-16, 1.000000000000000000 ) ) ;
#12723=CARTESIAN_POINT ( 'NONE',  ( 447.3372781065085633, 370.0000000000043769, 113.5502958579838122 ) ) ;
#12742=CARTESIAN_POINT ( 'NONE',  ( -439.4229916354183842, 394.9999999999955094, 96.05029585799300662 ) ) ;
#12748=ORIENTED_EDGE ( 'NONE', *, *, #34428, .T. ) ;
#12752=( BOUNDED_CURVE ( )  B_SPLINE_CURVE ( 3, ( #20410, #41877, #58051, #67250 ),
 .UNSPECIFIED., .F., .F. ) 
 B_SPLINE_CURVE_WITH_KNOTS ( ( 4, 4 ),
 ( 1.570796326794905440, 3.141592653589794004 ),
 .UNSPECIFIED. ) 
 CURVE ( )  GEOMETRIC_REPRESENTATION_ITEM ( )  RATIONAL_B_SPLINE_CURVE ( ( 1.000000000000000000, 0.8047378541243668248, 0.8047378541243668248, 1.000000000000000000 ) ) 
 REPRESENTATION_ITEM ( '' )  );
#12766=EDGE_CURVE ( 'NONE', #2857, #3113, #37314, .T. ) ;
#12810=LINE ( 'NONE', #1918, #36419 ) ;
#12865=CARTESIAN_POINT ( 'NONE',  ( -422.6627218934913230, 1.665334536937734811E-13, 108.5502958579881749 ) ) ;
#12872=LINE ( 'NONE', #67381, #29833 ) ;
#12874=DIRECTION ( 'NONE',  ( 1.000000000000000000, 1.387778780781445676E-16, 0.000000000000000000 ) ) ;
#12890=( GEOMETRIC_REPRESENTATION_CONTEXT ( 3 ) GLOBAL_UNCERTAINTY_ASSIGNED_CONTEXT ( ( #45856 ) ) GLOBAL_UNIT_ASSIGNED_CONTEXT ( ( #67079, #13588, #18869 ) ) REPRESENTATION_CONTEXT ( 'NONE', 'WORKASPACE' ) );
#12896=EDGE_LOOP ( 'NONE', ( #41554, #46784, #22278, #37922 ) ) ;
#12902=DIRECTION ( 'NONE',  ( 1.000000000000000000, 1.387778780781445676E-16, -1.110223024625156294E-16 ) ) ;
#12930=CIRCLE ( 'NONE', #35366, 5.000000000000004441 ) ;
#12955=ORIENTED_EDGE ( 'NONE', *, *, #42458, .F. ) ;
#13004=VECTOR ( 'NONE', #11626, 1000.000000000000000 ) ;
#13028=ORIENTED_EDGE ( 'NONE', *, *, #66972, .T. ) ;
#13081=CARTESIAN_POINT ( 'NONE',  ( 445.3372781065086201, 217.8591479523844612, 78.55029585798806124 ) ) ;
#13095=CARTESIAN_POINT ( 'NONE',  ( 442.3372781065083359, 370.0000000000043769, 108.5502958579838833 ) ) ;
#13106=VERTEX_POINT ( 'NONE', #55502 ) ;
#13108=ORIENTED_EDGE ( 'NONE', *, *, #14132, .F. ) ;
#13162=CARTESIAN_POINT ( 'NONE',  ( -442.6627218934916641, 394.9999999999954525, 103.5502958579924808 ) ) ;
#13189=CARTESIAN_POINT ( 'NONE',  ( -449.7337897053567417, 364.9999999999997726, 110.6213636698531673 ) ) ;
#13200=EDGE_CURVE ( 'NONE', #42554, #51645, #17871, .T. ) ;
#13234=DIRECTION ( 'NONE',  ( 0.000000000000000000, 6.779273404243065824E-32, -1.000000000000000000 ) ) ;
#13264=DIRECTION ( 'NONE',  ( 1.110223024625158749E-14, 0.000000000000000000, 1.000000000000000000 ) ) ;
#13269=AXIS2_PLACEMENT_3D ( 'NONE', #60677, #23411, #61371 ) ;
#13295=ORIENTED_EDGE ( 'NONE', *, *, #45343, .T. ) ;
#13298=EDGE_CURVE ( 'NONE', #33778, #7569, #11116, .T. ) ;
#13302=ORIENTED_EDGE ( 'NONE', *, *, #20071, .T. ) ;
#13320=VERTEX_POINT ( 'NONE', #14166 ) ;
#13323=( NAMED_UNIT ( * ) SI_UNIT ( $, .STERADIAN. ) SOLID_ANGLE_UNIT ( ) );
#13335=VERTEX_POINT ( 'NONE', #29648 ) ;
#13356=DIRECTION ( 'NONE',  ( 3.557538378468060822E-20, 5.551115123125781470E-17, -1.000000000000000000 ) ) ;
#13413=ORIENTED_EDGE ( 'NONE', *, *, #47530, .T. ) ;
#13415=DIRECTION ( 'NONE',  ( 0.000000000000000000, 1.000000000000000000, 2.184185950696548891E-33 ) ) ;
#13432=ORIENTED_EDGE ( 'NONE', *, *, #5545, .T. ) ;
#13434=VERTEX_POINT ( 'NONE', #10597 ) ;
#13450=PLANE ( 'NONE',  #28793 ) ;
#13521=STYLED_ITEM ( 'NONE', ( #34784 ), #16860 ) ;
#13542=DIRECTION ( 'NONE',  ( 0.000000000000000000, 0.000000000000000000, -1.000000000000000000 ) ) ;
#13555=VECTOR ( 'NONE', #23103, 1000.000000000000114 ) ;
#13561=CARTESIAN_POINT ( 'NONE',  ( -439.4229916354183842, 400.0000000000065370, -128.9497041420121093 ) ) ;
#13570=CARTESIAN_POINT ( 'NONE',  ( -452.6627218934913230, 399.9999999999998863, 113.5502958579881749 ) ) ;
#13571=DIRECTION ( 'NONE',  ( 1.000000000000000000, 1.850550996349095901E-16, 1.228197773518735191E-20 ) ) ;
#13588=( NAMED_UNIT ( * ) PLANE_ANGLE_UNIT ( ) SI_UNIT ( $, .RADIAN. ) );
#13621=ORIENTED_EDGE ( 'NONE', *, *, #27861, .T. ) ;
#13626=CARTESIAN_POINT ( 'NONE',  ( 445.3372781065086201, 177.8591479523844612, 78.55029585798806124 ) ) ;
#13627=VECTOR ( 'NONE', #28297, 1000.000000000000114 ) ;
#13631=ADVANCED_FACE ( 'NONE', ( #1808 ), #45396, .T. ) ;
#13639=DIRECTION ( 'NONE',  ( -1.387778780781445922E-16, 1.000000000000000000, 1.232595164407830946E-32 ) ) ;
#13706=DIRECTION ( 'NONE',  ( 2.922263668027335568E-20, 1.000000000000000000, -5.551115123125781470E-17 ) ) ;
#13727=VECTOR ( 'NONE', #55212, 1000.000000000000000 ) ;
#13730=CIRCLE ( 'NONE', #3586, 5.000000000000004441 ) ;
#13778=VECTOR ( 'NONE', #2406, 1000.000000000000000 ) ;
#13788=VECTOR ( 'NONE', #1128, 1000.000000000000000 ) ;
#13791=VERTEX_POINT ( 'NONE', #54097 ) ;
#13807=CYLINDRICAL_SURFACE ( 'NONE', #45813, 5.000000000000004441 ) ;
#13811=ADVANCED_FACE ( 'NONE', ( #665 ), #37595, .F. ) ;
#13822=ORIENTED_EDGE ( 'NONE', *, *, #50107, .T. ) ;
#13841=VECTOR ( 'NONE', #37518, 1000.000000000000000 ) ;
#13842=DIRECTION ( 'NONE',  ( 0.7071067811865475727, 5.551115123125781470E-17, -0.7071067811865474617 ) ) ;
#13852=ADVANCED_FACE ( 'NONE', ( #59046 ), #32335, .T. ) ;
#13916=ORIENTED_EDGE ( 'NONE', *, *, #43957, .F. ) ;
#13917=ORIENTED_EDGE ( 'NONE', *, *, #56299, .F. ) ;
#13933=FACE_OUTER_BOUND ( 'NONE', #11688, .T. ) ;
#13956=ORIENTED_EDGE ( 'NONE', *, *, #22879, .T. ) ;
#13970=VECTOR ( 'NONE', #41325, 1000.000000000000000 ) ;
#13975=VERTEX_POINT ( 'NONE', #61498 ) ;
#13990=ORIENTED_EDGE ( 'NONE', *, *, #27366, .T. ) ;
#14002=LINE ( 'NONE', #35106, #51257 ) ;
#14028=DIRECTION ( 'NONE',  ( -0.7071067811865475727, -2.220446049250312341E-16, 0.7071067811865474617 ) ) ;
#14047=CARTESIAN_POINT ( 'NONE',  ( -452.6627218934913799, 399.9999999999953957, 113.5502958579925803 ) ) ;
#14078=DIRECTION ( 'NONE',  ( 1.387778780781445922E-16, -1.000000000000000000, -3.469446951953615421E-17 ) ) ;
#14099=CARTESIAN_POINT ( 'NONE',  ( 429.8372781065087338, 395.0000000000001137, -123.9497041420121235 ) ) ;
#14132=EDGE_CURVE ( 'NONE', #68707, #66593, #17090, .T. ) ;
#14145=ADVANCED_FACE ( 'NONE', ( #22381 ), #16411, .F. ) ;
#14156=ORIENTED_EDGE ( 'NONE', *, *, #46473, .F. ) ;
#14162=PLANE ( 'NONE',  #46178 ) ;
#14166=CARTESIAN_POINT ( 'NONE',  ( -442.6627218934912662, 394.9999999999998295, 99.85872701201111568 ) ) ;
#14174=VERTEX_POINT ( 'NONE', #17447 ) ;
#14183=VECTOR ( 'NONE', #352, 1000.000000000000114 ) ;
#14197=UNCERTAINTY_MEASURE_WITH_UNIT (LENGTH_MEASURE( 1.000000000000000082E-05 ), #36592, 'distance_accuracy_value', 'NONE');
#14198=PLANE ( 'NONE',  #21656 ) ;
#14222=AXIS2_PLACEMENT_3D ( 'NONE', #16141, #37593, #65029 ) ;
#14230=EDGE_CURVE ( 'NONE', #56059, #46924, #17815, .T. ) ;
#14239=SURFACE_STYLE_FILL_AREA ( #43929 ) ;
#14267=DIRECTION ( 'NONE',  ( 1.387778780781445429E-16, -1.000000000000000000, -3.081487911019577365E-33 ) ) ;
#14295=EDGE_CURVE ( 'NONE', #46683, #43624, #67606, .T. ) ;
#14306=EDGE_CURVE ( 'NONE', #40455, #34795, #30104, .T. ) ;
#14320=VECTOR ( 'NONE', #62307, 1000.000000000000000 ) ;
#14328=AXIS2_PLACEMENT_3D ( 'NONE', #2958, #24757, #35306 ) ;
#14356=ORIENTED_EDGE ( 'NONE', *, *, #31094, .F. ) ;
#14358=FILL_AREA_STYLE_COLOUR ( '', #9409 ) ;
#14362=DIRECTION ( 'NONE',  ( 1.000000000000000000, 1.387778780781445429E-16, 0.000000000000000000 ) ) ;
#14385=ADVANCED_FACE ( 'NONE', ( #41684 ), #25865, .T. ) ;
#14391=FACE_OUTER_BOUND ( 'NONE', #17908, .T. ) ;
#14399=ORIENTED_EDGE ( 'NONE', *, *, #62080, .F. ) ;
#14440=ORIENTED_EDGE ( 'NONE', *, *, #25257, .F. ) ;
#14455=EDGE_CURVE ( 'NONE', #57503, #50950, #63489, .T. ) ;
#14468=EDGE_CURVE ( 'NONE', #16629, #67458, #11048, .T. ) ;
#14471=ORIENTED_EDGE ( 'NONE', *, *, #18798, .F. ) ;
#14518=AXIS2_PLACEMENT_3D ( 'NONE', #43230, #33752, #40104 ) ;
#14560=CARTESIAN_POINT ( 'NONE',  ( -422.6627218934914936, 399.9999999999998863, -146.4497041420118251 ) ) ;
#14572=DIRECTION ( 'NONE',  ( -3.081487911019579554E-32, -1.000000000000000000, -3.469446951953612956E-17 ) ) ;
#14576=ORIENTED_EDGE ( 'NONE', *, *, #11489, .T. ) ;
#14592=DIRECTION ( 'NONE',  ( 2.921639538487254261E-16, 1.134144525784205431E-35, 1.000000000000000000 ) ) ;
#14593=PLANE ( 'NONE',  #30912 ) ;
#14606=ORIENTED_EDGE ( 'NONE', *, *, #14455, .F. ) ;
#14626=CARTESIAN_POINT ( 'NONE',  ( 417.3372781065086201, 399.9999999999998863, 113.5502958579881891 ) ) ;
#14647=ORIENTED_EDGE ( 'NONE', *, *, #37476, .T. ) ;
#14676=CARTESIAN_POINT ( 'NONE',  ( -450.6627218934913230, 217.8591479523843475, -111.4497041420117966 ) ) ;
#14681=CARTESIAN_POINT ( 'NONE',  ( 445.3372781065086201, 217.8591479523844612, 78.55029585798806124 ) ) ;
#14697=CARTESIAN_POINT ( 'NONE',  ( -447.6627218934912662, 369.9999999999998295, 113.5502958579880328 ) ) ;
#14707=FILL_AREA_STYLE ('',( #4838 ) ) ;
#14734=EDGE_LOOP ( 'NONE', ( #19199, #31051, #17911, #33153 ) ) ;
#14752=EDGE_CURVE ( 'NONE', #9108, #66548, #3289, .T. ) ;
#14753=CARTESIAN_POINT ( 'NONE',  ( -447.6627218934913230, 399.9999999999997726, 83.55029585798818914 ) ) ;
#14757=CARTESIAN_POINT ( 'NONE',  ( 444.4083459183740956, 365.0000000000001137, -143.5207719538773006 ) ) ;
#14787=ORIENTED_EDGE ( 'NONE', *, *, #4617, .T. ) ;
#14812=ORIENTED_EDGE ( 'NONE', *, *, #29371, .T. ) ;
#14838=CLOSED_SHELL ( 'NONE', ( #11485, #21512, #53202, #27130, #13811, #16297 ) ) ;
#14860=DIRECTION ( 'NONE',  ( 1.387778780781445676E-16, -1.000000000000000000, -4.294171409582122931E-32 ) ) ;
#14868=ORIENTED_EDGE ( 'NONE', *, *, #12499, .F. ) ;
#14923=ADVANCED_FACE ( 'NONE', ( #23189 ), #62197, .F. ) ;
#14934=VECTOR ( 'NONE', #19472, 1000.000000000000000 ) ;
#14937=EDGE_LOOP ( 'NONE', ( #40297, #12748, #25724, #2583 ) ) ;
#14963=CYLINDRICAL_SURFACE ( 'NONE', #24196, 5.000000000000004441 ) ;
#15002=ORIENTED_EDGE ( 'NONE', *, *, #23735, .F. ) ;
#15008=EDGE_CURVE ( 'NONE', #32748, #33778, #9670, .T. ) ;
#15022=VERTEX_POINT ( 'NONE', #34451 ) ;
#15045=SURFACE_SIDE_STYLE ('',( #25949 ) ) ;
#15056=ORIENTED_EDGE ( 'NONE', *, *, #64905, .F. ) ;
#15070=ORIENTED_EDGE ( 'NONE', *, *, #7117, .F. ) ;
#15087=VECTOR ( 'NONE', #42298, 1000.000000000000000 ) ;
#15106=ORIENTED_EDGE ( 'NONE', *, *, #10089, .F. ) ;
#15124=VERTEX_POINT ( 'NONE', #595 ) ;
#15126=LINE ( 'NONE', #31641, #41953 ) ;
#15130=FILL_AREA_STYLE_COLOUR ( '', #32726 ) ;
#15140=EDGE_LOOP ( 'NONE', ( #58398, #500, #43053, #26877, #16134 ) ) ;
#15184=ORIENTED_EDGE ( 'NONE', *, *, #61694, .F. ) ;
#15196=CARTESIAN_POINT ( 'NONE',  ( -452.6627218934914367, 399.9999999999998863, -146.4497041420118251 ) ) ;
#15214=LINE ( 'NONE', #36678, #58015 ) ;
#15221=VECTOR ( 'NONE', #8095, 1000.000000000000000 ) ;
#15235=FACE_OUTER_BOUND ( 'NONE', #3424, .T. ) ;
#15236=PLANE ( 'NONE',  #49769 ) ;
#15241=VECTOR ( 'NONE', #27545, 1000.000000000000000 ) ;
#15246=DIRECTION ( 'NONE',  ( -1.387778780781446169E-16, 1.000000000000000000, 3.469446951953615421E-17 ) ) ;
#15251=CARTESIAN_POINT ( 'NONE',  ( -439.4229916354182706, 400.0000000000065370, -123.9497041420119530 ) ) ;
#15256=ORIENTED_EDGE ( 'NONE', *, *, #58508, .F. ) ;
#15297=DIRECTION ( 'NONE',  ( -0.000000000000000000, -1.000000000000000000, -0.000000000000000000 ) ) ;
#15303=CARTESIAN_POINT ( 'NONE',  ( 447.3372781065085064, 400.0000000000037517, 113.5502958579882034 ) ) ;
#15308=FILL_AREA_STYLE_COLOUR ( '', #55488 ) ;
#15320=CARTESIAN_POINT ( 'NONE',  ( -447.6627218934914936, 392.9289321881341266, -141.4497041420118251 ) ) ;
#15323=EDGE_CURVE ( 'NONE', #8527, #32748, #18866, .T. ) ;
#15343=EDGE_CURVE ( 'NONE', #63326, #34523, #33664, .T. ) ;
#15354=VERTEX_POINT ( 'NONE', #49815 ) ;
#15360=ORIENTED_EDGE ( 'NONE', *, *, #20391, .F. ) ;
#15383=LINE ( 'NONE', #48065, #25106 ) ;
#15419=LINE ( 'NONE', #37554, #43458 ) ;
#15421=CIRCLE ( 'NONE', #37907, 5.000000000000004441 ) ;
#15430=AXIS2_PLACEMENT_3D ( 'NONE', #9261, #4340, #45860 ) ;
#15435=EDGE_CURVE ( 'NONE', #28106, #59106, #20574, .T. ) ;
#15436=ADVANCED_FACE ( 'NONE', ( #30803 ), #42038, .T. ) ;
#15454=LINE ( 'NONE', #42177, #35460 ) ;
#15469=DIRECTION ( 'NONE',  ( 0.000000000000000000, 0.000000000000000000, -1.000000000000000000 ) ) ;
#15489=EDGE_CURVE ( 'NONE', #39831, #35076, #21959, .T. ) ;
#15496=CIRCLE ( 'NONE', #48004, 5.000000000000004441 ) ;
#15515=EDGE_CURVE ( 'NONE', #59605, #42064, #38856, .T. ) ;
#15519=DIRECTION ( 'NONE',  ( 1.850169831522831466E-16, -1.000000000000000000, 5.551115123125781470E-17 ) ) ;
#15562=FACE_OUTER_BOUND ( 'NONE', #51519, .T. ) ;
#15568=ORIENTED_EDGE ( 'NONE', *, *, #53429, .F. ) ;
#15575=EDGE_CURVE ( 'NONE', #7569, #26944, #16833, .T. ) ;
#15595=CARTESIAN_POINT ( 'NONE',  ( 437.3372781065085633, 400.0000000000000568, -136.4497041420118251 ) ) ;
#15602=VERTEX_POINT ( 'NONE', #26868 ) ;
#15620=LINE ( 'NONE', #64146, #23073 ) ;
#15634=ADVANCED_FACE ( 'NONE', ( #1891 ), #12432, .F. ) ;
#15649=( NAMED_UNIT ( * ) PLANE_ANGLE_UNIT ( ) SI_UNIT ( $, .RADIAN. ) );
#15656=CARTESIAN_POINT ( 'NONE',  ( 112.3013380801406385, 400.0000000000077307, 96.05029585798746439 ) ) ;
#15720=CARTESIAN_POINT ( 'NONE',  ( 442.3372781065085064, 390.0000000000001137, -146.4497041420117966 ) ) ;
#15754=CARTESIAN_POINT ( 'NONE',  ( 437.3372781065085633, 395.0000000000001137, -136.4497041420117966 ) ) ;
#15760=FACE_OUTER_BOUND ( 'NONE', #48289, .T. ) ;
#15788=ADVANCED_FACE ( 'NONE', ( #63735 ), #14162, .T. ) ;
#15806=ORIENTED_EDGE ( 'NONE', *, *, #48705, .T. ) ;
#15811=EDGE_CURVE ( 'NONE', #29891, #47734, #21843, .T. ) ;
#15818=EDGE_CURVE ( 'NONE', #12220, #48080, #37326, .T. ) ;
#15864=EDGE_CURVE ( 'NONE', #41137, #51945, #48213, .T. ) ;
#15922=FACE_OUTER_BOUND ( 'NONE', #61727, .T. ) ;
#15927=AXIS2_PLACEMENT_3D ( 'NONE', #68696, #15246, #41972 ) ;
#15942=FACE_OUTER_BOUND ( 'NONE', #5480, .T. ) ;
#15943=CARTESIAN_POINT ( 'NONE',  ( 437.3372781065084496, 395.0000000000043201, 103.5502958579839259 ) ) ;
#15951=LINE ( 'NONE', #31786, #46616 ) ;
#16003=LINE ( 'NONE', #29513, #43932 ) ;
#16064=LINE ( 'NONE', #64605, #13841 ) ;
#16075=VECTOR ( 'NONE', #43651, 1000.000000000000000 ) ;
#16116=DIRECTION ( 'NONE',  ( -1.000000000000000000, -1.850474763383843014E-16, 1.697708136181793677E-16 ) ) ;
#16134=ORIENTED_EDGE ( 'NONE', *, *, #3096, .F. ) ;
#16141=CARTESIAN_POINT ( 'NONE',  ( 112.3013380801408658, 388.0000000000065938, -123.9497041420121235 ) ) ;
#16154=CARTESIAN_POINT ( 'NONE',  ( 0.000000000000000000, 0.000000000000000000, 111.5502958579881749 ) ) ;
#16159=EDGE_CURVE ( 'NONE', #15124, #16476, #38552, .T. ) ;
#16182=DIRECTION ( 'NONE',  ( 1.387778780781445922E-16, -1.000000000000000000, -1.232595164407830946E-32 ) ) ;
#16183=VECTOR ( 'NONE', #30927, 1000.000000000000000 ) ;
#16210=VECTOR ( 'NONE', #54709, 1000.000000000000000 ) ;
#16221=DIRECTION ( 'NONE',  ( 0.000000000000000000, 0.000000000000000000, 1.000000000000000000 ) ) ;
#16240=CARTESIAN_POINT ( 'NONE',  ( 429.8372781065085633, 400.0000000000109708, 96.05029585798436642 ) ) ;
#16250=EDGE_CURVE ( 'NONE', #62318, #59386, #42707, .T. ) ;
#16268=ORIENTED_EDGE ( 'NONE', *, *, #8130, .T. ) ;
#16282=VECTOR ( 'NONE', #11706, 999.9999999999998863 ) ;
#16297=ADVANCED_FACE ( 'NONE', ( #59914 ), #16324, .T. ) ;
#16304=CARTESIAN_POINT ( 'NONE',  ( 447.3372781065086201, 400.0000000000044338, 113.5502958579838122 ) ) ;
#16324=PLANE ( 'NONE',  #19259 ) ;
#16356=CARTESIAN_POINT ( 'NONE',  ( 429.8372781065087906, 395.0000000000066507, -133.9497041420121377 ) ) ;
#16371=PLANE ( 'NONE',  #32333 ) ;
#16378=VECTOR ( 'NONE', #27514, 1000.000000000000000 ) ;
#16379=DIRECTION ( 'NONE',  ( -1.000000000000000000, -1.387778780781445922E-16, 0.000000000000000000 ) ) ;
#16392=VERTEX_POINT ( 'NONE', #7530 ) ;
#16395=CARTESIAN_POINT ( 'NONE',  ( 442.3372781065089612, 390.0000000000074465, -141.4497041420121377 ) ) ;
#16411=PLANE ( 'NONE',  #18021 ) ;
#16418=VECTOR ( 'NONE', #8890, 1000.000000000000000 ) ;
#16435=DIRECTION ( 'NONE',  ( 1.337618101958020291E-16, 0.000000000000000000, -1.000000000000000000 ) ) ;
#16444=ADVANCED_FACE ( 'NONE', ( #20143 ), #63752, .F. ) ;
#16448=CARTESIAN_POINT ( 'NONE',  ( -452.6627218934912662, 369.9999999999998295, 113.5502958579880328 ) ) ;
#16476=VERTEX_POINT ( 'NONE', #52499 ) ;
#16493=EDGE_CURVE ( 'NONE', #34795, #49146, #41109, .T. ) ;
#16496=CARTESIAN_POINT ( 'NONE',  ( 417.3372781065085633, 400.0000000000000568, -146.4497041420118251 ) ) ;
#16517=VECTOR ( 'NONE', #62195, 1000.000000000000000 ) ;
#16524=MANIFOLD_SOLID_BREP ( 'Boss-Extrude4', #14838 ) ;
#16550=CARTESIAN_POINT ( 'NONE',  ( -452.6627218934912094, 399.9999999999998295, 113.5502958579882602 ) ) ;
#16561=DIRECTION ( 'NONE',  ( -1.000000000000000000, 9.109522253334613014E-16, 1.697894969632811141E-16 ) ) ;
#16568=DIRECTION ( 'NONE',  ( -1.000000000000000000, 1.232595164407830946E-32, 7.703719777548943412E-34 ) ) ;
#16629=VERTEX_POINT ( 'NONE', #40138 ) ;
#16663=EDGE_LOOP ( 'NONE', ( #35157, #62200, #1465, #48632, #20623, #41173, #55680 ) ) ;
#16691=DIRECTION ( 'NONE',  ( 1.850550996349095901E-16, -1.000000000000000000, 5.551115123125781470E-17 ) ) ;
#16696=LINE ( 'NONE', #21626, #6891 ) ;
#16718=ORIENTED_EDGE ( 'NONE', *, *, #63160, .T. ) ;
#16744=MANIFOLD_SOLID_BREP ( 'Angle iron 35 X 35 X 5(4)', #23850 ) ;
#16773=EDGE_CURVE ( 'NONE', #13106, #63883, #37606, .T. ) ;
#16800=ORIENTED_EDGE ( 'NONE', *, *, #5234, .F. ) ;
#16803=EDGE_CURVE ( 'NONE', #29332, #45699, #59974, .T. ) ;
#16825=LINE ( 'NONE', #38286, #66869 ) ;
#16833=( BOUNDED_CURVE ( )  B_SPLINE_CURVE ( 3, ( #50094, #28279, #66633, #13162 ),
 .UNSPECIFIED., .F., .F. ) 
 B_SPLINE_CURVE_WITH_KNOTS ( ( 4, 4 ),
 ( 2.394390999492760841E-14, 1.570796326794902997 ),
 .UNSPECIFIED. ) 
 CURVE ( )  GEOMETRIC_REPRESENTATION_ITEM ( )  RATIONAL_B_SPLINE_CURVE ( ( 1.000000000000000000, 0.8047378541243690453, 0.8047378541243690453, 1.000000000000000000 ) ) 
 REPRESENTATION_ITEM ( '' )  );
#16838=PLANE ( 'NONE',  #403 ) ;
#16860=MANIFOLD_SOLID_BREP ( 'Angle iron 35 X 35 X 5(5)', #59713 ) ;
#16871=ORIENTED_EDGE ( 'NONE', *, *, #11540, .F. ) ;
#16877=FACE_OUTER_BOUND ( 'NONE', #27609, .T. ) ;
#16878=LINE ( 'NONE', #53117, #14183 ) ;
#16884=EDGE_CURVE ( 'NONE', #46731, #17356, #67154, .T. ) ;
#16908=ORIENTED_EDGE ( 'NONE', *, *, #10558, .F. ) ;
#16924=CARTESIAN_POINT ( 'NONE',  ( -417.6627218934913230, 399.9999999999997726, 113.5502958579881891 ) ) ;
#16965=CARTESIAN_POINT ( 'NONE',  ( 433.3728120124415568, 388.0000000000110276, 99.58582976391704733 ) ) ;
#16969=EDGE_CURVE ( 'NONE', #31046, #54939, #60461, .T. ) ;
#16978=AXIS2_PLACEMENT_3D ( 'NONE', #38721, #60167, #11986 ) ;
#16988=VERTEX_POINT ( 'NONE', #55173 ) ;
#16993=CARTESIAN_POINT ( 'NONE',  ( 412.3372781065085633, 179.4906275429376024, -146.4497041420117682 ) ) ;
#17020=DIRECTION ( 'NONE',  ( 1.387778780781446169E-16, -1.000000000000000000, -3.469446951953615421E-17 ) ) ;
#17027=CARTESIAN_POINT ( 'NONE',  ( -443.8104064242511413, 394.8690347851185152, -131.3748745853282287 ) ) ;
#17031=VECTOR ( 'NONE', #5416, 999.9999999999998863 ) ;
#17032=MECHANICAL_DESIGN_GEOMETRIC_PRESENTATION_REPRESENTATION('',(#67622),#27126);
#17033=EDGE_LOOP ( 'NONE', ( #11052, #18161, #35926, #18037, #24687, #38998, #33546 ) ) ;
#17042=CARTESIAN_POINT ( 'NONE',  ( 437.3372781065085633, 400.0000000000000568, -141.4497041420118251 ) ) ;
#17044=ADVANCED_FACE ( 'NONE', ( #60799 ), #66112, .F. ) ;
#17049=VERTEX_POINT ( 'NONE', #4492 ) ;
#17065=CARTESIAN_POINT ( 'NONE',  ( -450.6627218934913230, 217.8591479523843475, -111.4497041420117966 ) ) ;
#17081=ORIENTED_EDGE ( 'NONE', *, *, #67499, .F. ) ;
#17082=ORIENTED_EDGE ( 'NONE', *, *, #21130, .T. ) ;
#17090=LINE ( 'NONE', #10781, #28050 ) ;
#17107=ORIENTED_EDGE ( 'NONE', *, *, #20071, .F. ) ;
#17115=ORIENTED_EDGE ( 'NONE', *, *, #13200, .F. ) ;
#17130=EDGE_CURVE ( 'NONE', #19443, #13106, #47384, .T. ) ;
#17153=EDGE_CURVE ( 'NONE', #35973, #65355, #25953, .T. ) ;
#17189=CARTESIAN_POINT ( 'NONE',  ( 433.3728120124416137, 400.0000000000066507, 99.58582976392122532 ) ) ;
#17195=ORIENTED_EDGE ( 'NONE', *, *, #11489, .F. ) ;
#17211=ADVANCED_FACE ( 'NONE', ( #6117 ), #9775, .T. ) ;
#17221=CARTESIAN_POINT ( 'NONE',  ( 447.3372781065085064, 400.0000000000001137, -146.4497041420118535 ) ) ;
#17223=CARTESIAN_POINT ( 'NONE',  ( 447.3372781065085633, 400.0000000000000568, -111.4497041420118251 ) ) ;
#17272=CARTESIAN_POINT ( 'NONE',  ( -444.4229916354186116, 394.6798985497181889, 95.69015420990594123 ) ) ;
#17276=DIRECTION ( 'NONE',  ( 1.000000000000000000, 1.110223024625155594E-14, -1.110223024625155594E-14 ) ) ;
#17315=DIRECTION ( 'NONE',  ( 1.000000000000000000, 1.850550996349095901E-16, 1.228197773518735191E-20 ) ) ;
#17323=LINE ( 'NONE', #38798, #19808 ) ;
#17326=ORIENTED_EDGE ( 'NONE', *, *, #15864, .T. ) ;
#17341=CARTESIAN_POINT ( 'NONE',  ( 437.3372781065085633, 399.9999999999998863, 103.5502958579881891 ) ) ;
#17356=VERTEX_POINT ( 'NONE', #18084 ) ;
#17361=EDGE_CURVE ( 'NONE', #9937, #28396, #59573, .T. ) ;
#17372=DIRECTION ( 'NONE',  ( -1.000000000000000000, -1.110223024625155594E-14, 1.110223024625155594E-14 ) ) ;
#17389=VECTOR ( 'NONE', #12285, 1000.000000000000000 ) ;
#17392=VERTEX_POINT ( 'NONE', #18774 ) ;
#17447=CARTESIAN_POINT ( 'NONE',  ( 442.3372781065086201, 0.000000000000000000, -136.4497041420118251 ) ) ;
#17487=CARTESIAN_POINT ( 'NONE',  ( -417.6627218934913230, 397.0710678118653618, -111.4497041420117824 ) ) ;
#17525=DIRECTION ( 'NONE',  ( 0.7071067811865475727, 0.000000000000000000, 0.7071067811865474617 ) ) ;
#17566=VERTEX_POINT ( 'NONE', #32091 ) ;
#17599=CARTESIAN_POINT ( 'NONE',  ( 442.3372781065085633, 369.9999999999999432, 108.5502958579885870 ) ) ;
#17601=CYLINDRICAL_SURFACE ( 'NONE', #28581, 5.000000000000004441 ) ;
#17626=CYLINDRICAL_SURFACE ( 'NONE', #6955, 5.000000000000004441 ) ;
#17627=ADVANCED_FACE ( 'NONE', ( #8140 ), #29583, .T. ) ;
#17658=EDGE_CURVE ( 'NONE', #366, #66548, #7797, .T. ) ;
#17668=CARTESIAN_POINT ( 'NONE',  ( -450.6627218934913230, 177.8591479523843475, 78.55029585798814651 ) ) ;
#17714=CYLINDRICAL_SURFACE ( 'NONE', #64840, 5.000000000000170530 ) ;
#17720=DIRECTION ( 'NONE',  ( 1.000000000000000000, 1.748184826783646563E-16, 0.000000000000000000 ) ) ;
#17721=ORIENTED_EDGE ( 'NONE', *, *, #66260, .T. ) ;
#17744=UNCERTAINTY_MEASURE_WITH_UNIT (LENGTH_MEASURE( 1.000000000000000082E-05 ), #46815, 'distance_accuracy_value', 'NONE');
#17777=CARTESIAN_POINT ( 'NONE',  ( -447.6627218934912662, 389.9999999999998295, 113.5502958579881465 ) ) ;
#17781=ADVANCED_FACE ( 'NONE', ( #47478 ), #69291, .T. ) ;
#17795=ORIENTED_EDGE ( 'NONE', *, *, #28573, .F. ) ;
#17804=VERTEX_POINT ( 'NONE', #43234 ) ;
#17808=MANIFOLD_SOLID_BREP ( 'Cut-Extrude1[3]', #67631 ) ;
#17815=LINE ( 'NONE', #40302, #46079 ) ;
#17819=ORIENTED_EDGE ( 'NONE', *, *, #7117, .T. ) ;
#17862=ORIENTED_EDGE ( 'NONE', *, *, #52723, .F. ) ;
#17871=CIRCLE ( 'NONE', #53788, 5.000000000000004441 ) ;
#17885=CIRCLE ( 'NONE', #4384, 5.000000000000004441 ) ;
#17901=CARTESIAN_POINT ( 'NONE',  ( -452.6627218934913230, 399.9999999999998295, 113.5502958579881465 ) ) ;
#17908=EDGE_LOOP ( 'NONE', ( #68565, #52422, #15256, #14576 ) ) ;
#17911=ORIENTED_EDGE ( 'NONE', *, *, #1652, .F. ) ;
#17917=DIRECTION ( 'NONE',  ( -1.000000000000000000, -1.001918046209079887E-14, 9.729495617646301779E-15 ) ) ;
#17926=PLANE ( 'NONE',  #11349 ) ;
#17940=LINE ( 'NONE', #22514, #67826 ) ;
#17972=ADVANCED_FACE ( 'NONE', ( #24076 ), #45519, .T. ) ;
#17996=CARTESIAN_POINT ( 'NONE',  ( -7.662721893488489755, 395.0000000000064801, 308.5502958579854180 ) ) ;
#18021=AXIS2_PLACEMENT_3D ( 'NONE', #21007, #26962, #42452 ) ;
#18022=CARTESIAN_POINT ( 'NONE',  ( -452.6627218934860366, 395.0000000000064801, -116.4497041420121377 ) ) ;
#18023=ORIENTED_EDGE ( 'NONE', *, *, #67996, .T. ) ;
#18034=EDGE_LOOP ( 'NONE', ( #31761, #19492, #64500, #278 ) ) ;
#18037=ORIENTED_EDGE ( 'NONE', *, *, #40758, .F. ) ;
#18047=LINE ( 'NONE', #49, #61033 ) ;
#18050=DIRECTION ( 'NONE',  ( 1.387778780781446169E-16, -1.000000000000000000, -3.469446951953615421E-17 ) ) ;
#18058=VECTOR ( 'NONE', #18971, 1000.000000000000000 ) ;
#18081=VERTEX_POINT ( 'NONE', #43246 ) ;
#18084=CARTESIAN_POINT ( 'NONE',  ( 112.3013380801406100, 400.0000000000077307, 91.05029585798746439 ) ) ;
#18086=CARTESIAN_POINT ( 'NONE',  ( 445.3372781065086201, 177.8591479523844612, 78.55029585798806124 ) ) ;
#18100=ADVANCED_FACE ( 'NONE', ( #64723 ), #66142, .T. ) ;
#18141=LINE ( 'NONE', #44523, #23114 ) ;
#18154=DIRECTION ( 'NONE',  ( 1.000000000000000000, -1.540743955509788682E-33, -1.110223024625156540E-16 ) ) ;
#18161=ORIENTED_EDGE ( 'NONE', *, *, #10155, .F. ) ;
#18168=FACE_OUTER_BOUND ( 'NONE', #23410, .T. ) ;
#18174=CARTESIAN_POINT ( 'NONE',  ( 442.3372781065086201, 395.0000000000043201, 108.5502958579839117 ) ) ;
#18188=DIRECTION ( 'NONE',  ( 1.020422603260505347E-14, -1.000000000000000000, -5.551115123125782702E-17 ) ) ;
#18190=FACE_OUTER_BOUND ( 'NONE', #66226, .T. ) ;
#18194=CARTESIAN_POINT ( 'NONE',  ( -439.4229916354185548, 388.0000000000064801, -133.9497041420121377 ) ) ;
#18198=DIRECTION ( 'NONE',  ( -7.703719777548945123E-34, -1.479221584281240009E-31, 1.000000000000000000 ) ) ;
#18210=VECTOR ( 'NONE', #61236, 1000.000000000000114 ) ;
#18212=ORIENTED_EDGE ( 'NONE', *, *, #24367, .T. ) ;
#18229=ORIENTED_EDGE ( 'NONE', *, *, #33056, .T. ) ;
#18236=CARTESIAN_POINT ( 'NONE',  ( 50.98853755884125860, 400.0000000000071054, 91.05029585798797598 ) ) ;
#18242=CARTESIAN_POINT ( 'NONE',  ( -447.6627218934918915, 367.0710678118718988, -141.4497041420121377 ) ) ;
#18259=CARTESIAN_POINT ( 'NONE',  ( 447.3372781065082791, 400.0000000000044338, 78.55029585798382641 ) ) ;
#18271=DIRECTION ( 'NONE',  ( 0.7071067811865476838, 1.110223024625156294E-16, 0.7071067811865474617 ) ) ;
#18298=ORIENTED_EDGE ( 'NONE', *, *, #65042, .F. ) ;
#18309=CARTESIAN_POINT ( 'NONE',  ( -452.6627218934913230, 400.0000000000000568, -146.4497041420117398 ) ) ;
#18329=CARTESIAN_POINT ( 'NONE',  ( -439.4229916354182706, 400.0000000000064801, 91.05029585798840230 ) ) ;
#18336=DIRECTION ( 'NONE',  ( -0.000000000000000000, -6.405132834375902056E-16, 1.000000000000000000 ) ) ;
#18354=VECTOR ( 'NONE', #11675, 1000.000000000000000 ) ;
#18364=EDGE_CURVE ( 'NONE', #28296, #29979, #46383, .T. ) ;
#18405=LINE ( 'NONE', #50420, #11791 ) ;
#18426=CYLINDRICAL_SURFACE ( 'NONE', #56970, 5.000000000000004441 ) ;
#18499=VECTOR ( 'NONE', #45598, 1000.000000000000000 ) ;
#18505=LINE ( 'NONE', #29069, #37427 ) ;
#18515=DIRECTION ( 'NONE',  ( -1.000000000000000000, -1.850550996349095901E-16, -1.228197773518735191E-20 ) ) ;
#18546=CARTESIAN_POINT ( 'NONE',  ( 447.3372781065086201, 217.8591479523844612, 78.55029585798806124 ) ) ;
#18570=CARTESIAN_POINT ( 'NONE',  ( -430.1627218934915504, 399.9999999999996021, 91.05029585798840230 ) ) ;
#18612=VECTOR ( 'NONE', #68065, 1000.000000000000000 ) ;
#18671=CARTESIAN_POINT ( 'NONE',  ( -442.6627218934914367, 399.9999999999998863, -141.4497041420118251 ) ) ;
#18679=DIRECTION ( 'NONE',  ( 0.000000000000000000, 3.469446951953616038E-17, -1.000000000000000000 ) ) ;
#18710=ORIENTED_EDGE ( 'NONE', *, *, #21537, .F. ) ;
#18774=CARTESIAN_POINT ( 'NONE',  ( 437.3372781065085633, 395.0000000000001137, -136.4497041420117966 ) ) ;
#18787=DIRECTION ( 'NONE',  ( -0.7071067811865476838, 0.000000000000000000, -0.7071067811865474617 ) ) ;
#18798=EDGE_CURVE ( 'NONE', #5564, #52445, #25994, .T. ) ;
#18801=CARTESIAN_POINT ( 'NONE',  ( 50.98853755884140782, 395.0000000000004547, 96.05029585798814651 ) ) ;
#18818=EDGE_CURVE ( 'NONE', #19443, #62318, #65340, .T. ) ;
#18844=ADVANCED_FACE ( 'NONE', ( #3316 ), #62755, .T. ) ;
#18845=VECTOR ( 'NONE', #55827, 1000.000000000000000 ) ;
#18866=LINE ( 'NONE', #18174, #13555 ) ;
#18869=( NAMED_UNIT ( * ) SI_UNIT ( $, .STERADIAN. ) SOLID_ANGLE_UNIT ( ) );
#18875=DIRECTION ( 'NONE',  ( -1.000000000000000000, -1.110223024625118675E-14, 1.110223024625118675E-14 ) ) ;
#18902=ORIENTED_EDGE ( 'NONE', *, *, #65042, .T. ) ;
#18920=CARTESIAN_POINT ( 'NONE',  ( -439.4229916354185548, 400.0000000000065370, -128.9497041420121093 ) ) ;
#18929=PLANE ( 'NONE',  #68154 ) ;
#18949=COLOUR_RGB ( '',0.7921568627450980005, 0.8196078431372548767, 0.9333333333333333481 ) ;
#18971=DIRECTION ( 'NONE',  ( -1.000000000000000000, -1.387778780781446415E-16, 0.000000000000000000 ) ) ;
#19007=VECTOR ( 'NONE', #44631, 1000.000000000000000 ) ;
#19044=CARTESIAN_POINT ( 'NONE',  ( -422.6627218934914936, 399.9999999999998863, -146.4497041420118251 ) ) ;
#19058=VERTEX_POINT ( 'NONE', #59521 ) ;
#19069=ADVANCED_FACE ( 'NONE', ( #64822 ), #27521, .T. ) ;
#19073=DIRECTION ( 'NONE',  ( 0.7071067811865474617, -5.551115123125781716E-16, 0.7071067811865475727 ) ) ;
#19137=LINE ( 'NONE', #40591, #32394 ) ;
#19199=ORIENTED_EDGE ( 'NONE', *, *, #43310, .T. ) ;
#19232=FACE_OUTER_BOUND ( 'NONE', #6807, .T. ) ;
#19259=AXIS2_PLACEMENT_3D ( 'NONE', #44083, #53935, #493 ) ;
#19288=CARTESIAN_POINT ( 'NONE',  ( 424.8372781065089612, 400.0000000000000568, -123.9497041420121235 ) ) ;
#19311=CARTESIAN_POINT ( 'NONE',  ( -422.6627218934912662, 399.9999999999998295, 113.5502958579882602 ) ) ;
#19319=DIRECTION ( 'NONE',  ( -0.7071067811865545671, 2.831068712794148784E-15, -0.7071067811865405783 ) ) ;
#19354=CARTESIAN_POINT ( 'NONE',  ( -452.6627218934913230, 1.665334536937734811E-13, 113.5502958579881749 ) ) ;
#19438=ORIENTED_EDGE ( 'NONE', *, *, #42540, .T. ) ;
#19443=VERTEX_POINT ( 'NONE', #51940 ) ;
#19456=ORIENTED_EDGE ( 'NONE', *, *, #47699, .T. ) ;
#19458=VECTOR ( 'NONE', #14028, 1000.000000000000114 ) ;
#19472=DIRECTION ( 'NONE',  ( 5.294909809750763265E-16, 1.000000000000000000, 1.110223024625156171E-16 ) ) ;
#19483=ADVANCED_FACE ( 'NONE', ( #19232 ), #32901, .F. ) ;
#19492=ORIENTED_EDGE ( 'NONE', *, *, #16493, .T. ) ;
#19497=CYLINDRICAL_SURFACE ( 'NONE', #69075, 5.000000000000004441 ) ;
#19511=DIRECTION ( 'NONE',  ( -1.000000000000000000, 0.000000000000000000, 0.000000000000000000 ) ) ;
#19517=ORIENTED_EDGE ( 'NONE', *, *, #14455, .T. ) ;
#19537=CARTESIAN_POINT ( 'NONE',  ( -452.6627218934913230, 1.665334536937734811E-13, 83.55029585798817493 ) ) ;
#19541=ORIENTED_EDGE ( 'NONE', *, *, #42231, .F. ) ;
#19556=DIRECTION ( 'NONE',  ( -9.729547286656084292E-15, -7.216449660064492742E-16, -1.000000000000000000 ) ) ;
#19564=AXIS2_PLACEMENT_3D ( 'NONE', #14047, #19319, #8787 ) ;
#19595=ORIENTED_EDGE ( 'NONE', *, *, #6848, .T. ) ;
#19611=EDGE_CURVE ( 'NONE', #57474, #7362, #61377, .T. ) ;
#19628=EDGE_CURVE ( 'NONE', #36796, #34795, #1592, .T. ) ;
#19658=AXIS2_PLACEMENT_3D ( 'NONE', #10322, #63458, #20197 ) ;
#19668=ORIENTED_EDGE ( 'NONE', *, *, #32181, .F. ) ;
#19709=EDGE_LOOP ( 'NONE', ( #23921, #58750, #12272, #239 ) ) ;
#19768=ORIENTED_EDGE ( 'NONE', *, *, #12162, .T. ) ;
#19784=DIRECTION ( 'NONE',  ( 1.387778780781445922E-16, -1.000000000000000000, -1.232595164407830946E-32 ) ) ;
#19795=DIRECTION ( 'NONE',  ( 1.387778780781446169E-16, -1.000000000000000000, -3.469446951953615421E-17 ) ) ;
#19808=VECTOR ( 'NONE', #53209, 1000.000000000000000 ) ;
#19821=UNCERTAINTY_MEASURE_WITH_UNIT (LENGTH_MEASURE( 1.000000000000000082E-05 ), #69363, 'distance_accuracy_value', 'NONE');
#19838=CARTESIAN_POINT ( 'NONE',  ( -452.6627218934914367, 399.9999999999998863, -146.4497041420118251 ) ) ;
#19839=ORIENTED_EDGE ( 'NONE', *, *, #37934, .T. ) ;
#19861=ORIENTED_EDGE ( 'NONE', *, *, #28252, .F. ) ;
#19875=LINE ( 'NONE', #41331, #21064 ) ;
#19920=DIRECTION ( 'NONE',  ( 1.000000000000000000, 1.850550996349095901E-16, 1.228197773518735191E-20 ) ) ;
#19924=CARTESIAN_POINT ( 'NONE',  ( 442.3372781065085633, 400.0000000000000568, -116.4497041420118393 ) ) ;
#19948=( BOUNDED_CURVE ( )  B_SPLINE_CURVE ( 3, ( #24917, #18242, #45678, #3120 ),
 .UNSPECIFIED., .F., .F. ) 
 B_SPLINE_CURVE_WITH_KNOTS ( ( 4, 4 ),
 ( 3.140184917367546882E-16, 1.570796326794896780 ),
 .UNSPECIFIED. ) 
 CURVE ( )  GEOMETRIC_REPRESENTATION_ITEM ( )  RATIONAL_B_SPLINE_CURVE ( ( 1.000000000000000000, 0.8047378541243649375, 0.8047378541243649375, 1.000000000000000000 ) ) 
 REPRESENTATION_ITEM ( '' )  );
#19972=FACE_OUTER_BOUND ( 'NONE', #21357, .T. ) ;
#19977=CARTESIAN_POINT ( 'NONE',  ( 112.3013380801408658, 400.0000000000066507, -123.9497041420121235 ) ) ;
#19994=ORIENTED_EDGE ( 'NONE', *, *, #67890, .T. ) ;
#19995=DIRECTION ( 'NONE',  ( 1.000000000000000000, 1.850550996349095901E-16, 1.228197773518735191E-20 ) ) ;
#20010=ORIENTED_EDGE ( 'NONE', *, *, #69155, .F. ) ;
#20041=LINE ( 'NONE', #14753, #15221 ) ;
#20071=EDGE_CURVE ( 'NONE', #24241, #34219, #13730, .T. ) ;
#20089=EDGE_CURVE ( 'NONE', #47734, #38085, #48663, .T. ) ;
#20104=ORIENTED_EDGE ( 'NONE', *, *, #56299, .T. ) ;
#20127=DIRECTION ( 'NONE',  ( 0.000000000000000000, 1.000000000000000000, 0.000000000000000000 ) ) ;
#20143=FACE_OUTER_BOUND ( 'NONE', #22508, .T. ) ;
#20145=CARTESIAN_POINT ( 'NONE',  ( -439.4229916354183842, 388.0000000000020464, 91.05029585799266556 ) ) ;
#20146=CIRCLE ( 'NONE', #48232, 5.000000000000170530 ) ;
#20184=CARTESIAN_POINT ( 'NONE',  ( -417.6627218934913230, 179.4906275429376308, -144.4497041420118819 ) ) ;
#20197=DIRECTION ( 'NONE',  ( -1.000000000000000000, 0.000000000000000000, 0.000000000000000000 ) ) ;
#20222=CARTESIAN_POINT ( 'NONE',  ( -452.6627218934912662, 364.9999999999998295, 113.5502958579879760 ) ) ;
#20227=CARTESIAN_POINT ( 'NONE',  ( 417.3372781065083359, 395.0000000000041496, 83.55029585798409641 ) ) ;
#20232=EDGE_CURVE ( 'NONE', #57073, #10801, #31286, .T. ) ;
#20257=VECTOR ( 'NONE', #25524, 1000.000000000000000 ) ;
#20262=ORIENTED_EDGE ( 'NONE', *, *, #30667, .T. ) ;
#20286=ORIENTED_EDGE ( 'NONE', *, *, #40501, .T. ) ;
#20295=ORIENTED_EDGE ( 'NONE', *, *, #47994, .T. ) ;
#20303=DIRECTION ( 'NONE',  ( 0.000000000000000000, -1.000000000000000000, -2.184185950696548891E-33 ) ) ;
#20326=FACE_OUTER_BOUND ( 'NONE', #59021, .T. ) ;
#20327=PRESENTATION_STYLE_ASSIGNMENT (( #47392 ) ) ;
#20337=LINE ( 'NONE', #29509, #19458 ) ;
#20391=EDGE_CURVE ( 'NONE', #47218, #22681, #23151, .T. ) ;
#20392=VERTEX_POINT ( 'NONE', #1342 ) ;
#20395=SURFACE_STYLE_USAGE ( .BOTH. , #3534 ) ;
#20396=DIRECTION ( 'NONE',  ( 1.850371928290090422E-16, -1.000000000000000000, -1.110223024625156294E-16 ) ) ;
#20410=CARTESIAN_POINT ( 'NONE',  ( 447.3372781065089612, 365.0000000000064233, -146.4497041420121377 ) ) ;
#20423=ORIENTED_EDGE ( 'NONE', *, *, #15515, .T. ) ;
#20452=CARTESIAN_POINT ( 'NONE',  ( -443.8115333961470128, 394.8687311169578606, -126.5269779445883387 ) ) ;
#20487=VERTEX_POINT ( 'NONE', #646 ) ;
#20504=CARTESIAN_POINT ( 'NONE',  ( -452.6627218934859798, 395.0000000000064801, -136.4497041420121661 ) ) ;
#20523=CARTESIAN_POINT ( 'NONE',  ( 112.3013380801406811, 400.0000000000077307, 101.0502958579874644 ) ) ;
#20538=ORIENTED_EDGE ( 'NONE', *, *, #43359, .T. ) ;
#20541=ORIENTED_EDGE ( 'NONE', *, *, #16159, .T. ) ;
#20546=EDGE_CURVE ( 'NONE', #23006, #41527, #65723, .T. ) ;
#20566=LINE ( 'NONE', #31479, #67785 ) ;
#20570=( NAMED_UNIT ( * ) SI_UNIT ( $, .STERADIAN. ) SOLID_ANGLE_UNIT ( ) );
#20574=LINE ( 'NONE', #51904, #5693 ) ;
#20598=ORIENTED_EDGE ( 'NONE', *, *, #49061, .T. ) ;
#20606=CARTESIAN_POINT ( 'NONE',  ( -419.7337897053564006, 395.0000000000001705, 80.62136366985323832 ) ) ;
#20613=CARTESIAN_POINT ( 'NONE',  ( 412.3372781065085633, 179.4906275429376024, -144.4497041420117682 ) ) ;
#20623=ORIENTED_EDGE ( 'NONE', *, *, #52639, .F. ) ;
#20631=EDGE_CURVE ( 'NONE', #51945, #17566, #52640, .T. ) ;
#20662=FACE_OUTER_BOUND ( 'NONE', #4988, .T. ) ;
#20702=VECTOR ( 'NONE', #44644, 1000.000000000000000 ) ;
#20707=VECTOR ( 'NONE', #3487, 1000.000000000000000 ) ;
#20721=CARTESIAN_POINT ( 'NONE',  ( 447.3372781065083927, 395.0000000000043769, 103.5502958579838264 ) ) ;
#20723=DIRECTION ( 'NONE',  ( -0.7071067811865473507, -1.232595164407830946E-32, 0.7071067811865476838 ) ) ;
#20729=ORIENTED_EDGE ( 'NONE', *, *, #1666, .T. ) ;
#20745=CARTESIAN_POINT ( 'NONE',  ( -452.6627218934913230, 399.9999999999997726, 113.5502958579881891 ) ) ;
#20781=ORIENTED_EDGE ( 'NONE', *, *, #18364, .F. ) ;
#20830=DIRECTION ( 'NONE',  ( 1.697894969632809662E-16, -1.110223024625155801E-16, 1.000000000000000000 ) ) ;
#20836=CARTESIAN_POINT ( 'NONE',  ( -440.1146514826276075, 388.0000000000064801, -133.9016337311480243 ) ) ;
#20845=CARTESIAN_POINT ( 'NONE',  ( 447.3372781065085633, 400.0000000000000568, -146.4497041420117966 ) ) ;
#20857=CARTESIAN_POINT ( 'NONE',  ( -422.6627218934914936, 394.9999999999956799, 83.55029585799226766 ) ) ;
#20867=VERTEX_POINT ( 'NONE', #69260 ) ;
#20885=LINE ( 'NONE', #25835, #568 ) ;
#20890=CARTESIAN_POINT ( 'NONE',  ( 417.3372781065086201, 399.9999999999998863, 108.5502958579882034 ) ) ;
#20903=CARTESIAN_POINT ( 'NONE',  ( -440.1146514826276643, 388.0000000000064801, -133.9016337311480243 ) ) ;
#20914=ORIENTED_EDGE ( 'NONE', *, *, #6659, .F. ) ;
#20922=ORIENTED_EDGE ( 'NONE', *, *, #67681, .F. ) ;
#20936=PLANE ( 'NONE',  #49968 ) ;
#20962=VERTEX_POINT ( 'NONE', #65733 ) ;
#20970=VERTEX_POINT ( 'NONE', #66092 ) ;
#20982=EDGE_CURVE ( 'NONE', #47734, #13320, #29134, .T. ) ;
#20989=AXIS2_PLACEMENT_3D ( 'NONE', #41441, #52334, #62896 ) ;
#21007=CARTESIAN_POINT ( 'NONE',  ( 447.3372781065085633, 400.0000000000000568, -146.4497041420118251 ) ) ;
#21018=FACE_OUTER_BOUND ( 'NONE', #8135, .T. ) ;
#21042=DIRECTION ( 'NONE',  ( 1.000000000000000000, 1.387778780781444936E-16, 0.000000000000000000 ) ) ;
#21053=DIRECTION ( 'NONE',  ( 0.000000000000000000, 1.000000000000000000, 2.184185950696548891E-33 ) ) ;
#21064=VECTOR ( 'NONE', #51541, 1000.000000000000000 ) ;
#21088=PRESENTATION_STYLE_ASSIGNMENT (( #5247 ) ) ;
#21102=CARTESIAN_POINT ( 'NONE',  ( 417.3372781065086201, 0.000000000000000000, -146.4497041420118251 ) ) ;
#21125=ORIENTED_EDGE ( 'NONE', *, *, #28010, .F. ) ;
#21130=EDGE_CURVE ( 'NONE', #41110, #14174, #8729, .T. ) ;
#21137=CARTESIAN_POINT ( 'NONE',  ( 442.3372781065085633, 390.0000000000001137, 108.5502958579883170 ) ) ;
#21182=CARTESIAN_POINT ( 'NONE',  ( -452.6627218934914936, 364.9999999999953957, 113.5502958579925945 ) ) ;
#21219=ADVANCED_FACE ( 'NONE', ( #19972 ), #3438, .T. ) ;
#21246=DIRECTION ( 'NONE',  ( -1.000000000000000000, 3.344045254895050726E-17, -1.337618101958020291E-16 ) ) ;
#21280=CARTESIAN_POINT ( 'NONE',  ( -439.4229916354183274, 388.0000000000020464, 101.0502958579930066 ) ) ;
#21311=DIRECTION ( 'NONE',  ( -1.850371928290090422E-16, 1.000000000000000000, 1.110223024625156171E-16 ) ) ;
#21328=VERTEX_POINT ( 'NONE', #10094 ) ;
#21334=VECTOR ( 'NONE', #41898, 1000.000000000000000 ) ;
#21357=EDGE_LOOP ( 'NONE', ( #9766, #43430, #29429, #40306 ) ) ;
#21410=ORIENTED_EDGE ( 'NONE', *, *, #788, .T. ) ;
#21432=CARTESIAN_POINT ( 'NONE',  ( 112.3013380801406669, 395.0000000000010800, 91.05029585798746439 ) ) ;
#21442=SURFACE_STYLE_USAGE ( .BOTH. , #60477 ) ;
#21449=EDGE_CURVE ( 'NONE', #52445, #22995, #23445, .T. ) ;
#21453=DIRECTION ( 'NONE',  ( 1.387778780781445429E-16, -1.000000000000000000, -3.081487911019577365E-33 ) ) ;
#21501=VECTOR ( 'NONE', #25333, 1000.000000000000000 ) ;
#21503=AXIS2_PLACEMENT_3D ( 'NONE', #11744, #33915, #64877 ) ;
#21512=ADVANCED_FACE ( 'NONE', ( #28713 ), #60710, .T. ) ;
#21523=ORIENTED_EDGE ( 'NONE', *, *, #51917, .F. ) ;
#21527=DIRECTION ( 'NONE',  ( -2.921639538487254261E-16, -1.134144525784205431E-35, -1.000000000000000000 ) ) ;
#21536=CARTESIAN_POINT ( 'NONE',  ( -452.6627218934913230, 399.9999999999998863, 113.5502958579881749 ) ) ;
#21537=EDGE_CURVE ( 'NONE', #43634, #66845, #12184, .T. ) ;
#21539=ORIENTED_EDGE ( 'NONE', *, *, #48256, .T. ) ;
#21547=VECTOR ( 'NONE', #35867, 1000.000000000000000 ) ;
#21559=VECTOR ( 'NONE', #30939, 1000.000000000000000 ) ;
#21577=ORIENTED_EDGE ( 'NONE', *, *, #61694, .T. ) ;
#21582=EDGE_CURVE ( 'NONE', #9188, #10959, #1275, .T. ) ;
#21592=ORIENTED_EDGE ( 'NONE', *, *, #39554, .F. ) ;
#21613=VERTEX_POINT ( 'NONE', #68422 ) ;
#21626=CARTESIAN_POINT ( 'NONE',  ( -417.6627218934913230, 219.4906275429376308, -144.4497041420118819 ) ) ;
#21636=VERTEX_POINT ( 'NONE', #57519 ) ;
#21652=VECTOR ( 'NONE', #27673, 1000.000000000000000 ) ;
#21656=AXIS2_PLACEMENT_3D ( 'NONE', #67329, #3631, #13842 ) ;
#21702=FACE_OUTER_BOUND ( 'NONE', #36586, .T. ) ;
#21708=AXIS2_PLACEMENT_3D ( 'NONE', #55111, #18188, #38595 ) ;
#21715=DIRECTION ( 'NONE',  ( -1.000000000000000000, -1.001918046209079887E-14, 9.729495617646301779E-15 ) ) ;
#21719=DIRECTION ( 'NONE',  ( 0.7071067811865475727, 2.220446049250312341E-16, -0.7071067811865474617 ) ) ;
#21724=ORIENTED_EDGE ( 'NONE', *, *, #69466, .F. ) ;
#21736=( GEOMETRIC_REPRESENTATION_CONTEXT ( 3 ) GLOBAL_UNCERTAINTY_ASSIGNED_CONTEXT ( ( #24061 ) ) GLOBAL_UNIT_ASSIGNED_CONTEXT ( ( #31232, #27310, #55087 ) ) REPRESENTATION_CONTEXT ( 'NONE', 'WORKASPACE' ) );
#21756=VECTOR ( 'NONE', #38755, 1000.000000000000114 ) ;
#21759=( NAMED_UNIT ( * ) SI_UNIT ( $, .STERADIAN. ) SOLID_ANGLE_UNIT ( ) );
#21765=( BOUNDED_CURVE ( )  B_SPLINE_CURVE ( 3, ( #69134, #54334, #20606, #42415 ),
 .UNSPECIFIED., .F., .F. ) 
 B_SPLINE_CURVE_WITH_KNOTS ( ( 4, 4 ),
 ( -2.664535259100375697E-15, 1.570796326794774433 ),
 .UNSPECIFIED. ) 
 CURVE ( )  GEOMETRIC_REPRESENTATION_ITEM ( )  RATIONAL_B_SPLINE_CURVE ( ( 1.000000000000000000, 0.8047378541243930261, 0.8047378541243930261, 1.000000000000000000 ) ) 
 REPRESENTATION_ITEM ( '' )  );
#21782=CYLINDRICAL_SURFACE ( 'NONE', #14518, 5.000000000000115463 ) ;
#21785=( NAMED_UNIT ( * ) PLANE_ANGLE_UNIT ( ) SI_UNIT ( $, .RADIAN. ) );
#21817=ORIENTED_EDGE ( 'NONE', *, *, #42935, .F. ) ;
#21831=DIRECTION ( 'NONE',  ( -1.000000000000000000, 0.000000000000000000, 0.000000000000000000 ) ) ;
#21843=LINE ( 'NONE', #33106, #58516 ) ;
#21906=CARTESIAN_POINT ( 'NONE',  ( 447.3372781065083927, 395.0000000000043769, 91.05029585798388325 ) ) ;
#21926=EDGE_LOOP ( 'NONE', ( #63329, #51842, #8160, #65619 ) ) ;
#21929=DIRECTION ( 'NONE',  ( -1.000000000000000000, 3.344045254895050726E-17, -1.337618101958020291E-16 ) ) ;
#21959=LINE ( 'NONE', #69103, #29269 ) ;
#21960=DIRECTION ( 'NONE',  ( 3.306261395983863330E-15, 1.000000000000000000, -5.551115123125782702E-17 ) ) ;
#21990=EDGE_CURVE ( 'NONE', #63860, #33355, #23184, .T. ) ;
#21992=ORIENTED_EDGE ( 'NONE', *, *, #16803, .F. ) ;
#22036=DIRECTION ( 'NONE',  ( -1.387778780781445676E-15, -2.095411779493312608E-31, -1.000000000000000000 ) ) ;
#22037=ORIENTED_EDGE ( 'NONE', *, *, #38249, .F. ) ;
#22046=VECTOR ( 'NONE', #12902, 1000.000000000000000 ) ;
#22068=DIRECTION ( 'NONE',  ( 1.110223024625158749E-14, 0.000000000000000000, 1.000000000000000000 ) ) ;
#22073=CARTESIAN_POINT ( 'NONE',  ( 112.3013380801407095, 388.0000000000077307, 91.05029585798746439 ) ) ;
#22118=ORIENTED_EDGE ( 'NONE', *, *, #59385, .T. ) ;
#22120=EDGE_LOOP ( 'NONE', ( #11083, #24345, #50636, #33255 ) ) ;
#22121=FACE_OUTER_BOUND ( 'NONE', #51642, .T. ) ;
#22132=VECTOR ( 'NONE', #21042, 1000.000000000000000 ) ;
#22160=VECTOR ( 'NONE', #11804, 1000.000000000000000 ) ;
#22245=AXIS2_PLACEMENT_3D ( 'NONE', #67094, #29778, #13264 ) ;
#22262=CARTESIAN_POINT ( 'NONE',  ( 447.3372781065086201, 0.000000000000000000, -146.4497041420118251 ) ) ;
#22272=DIRECTION ( 'NONE',  ( -1.000000000000000000, -1.387778780781448141E-16, 5.551115123125781716E-16 ) ) ;
#22278=ORIENTED_EDGE ( 'NONE', *, *, #47699, .F. ) ;
#22287=AXIS2_PLACEMENT_3D ( 'NONE', #22073, #48098, #27340 ) ;
#22296=CARTESIAN_POINT ( 'NONE',  ( 412.3372781065086201, 399.9999999999998863, 78.55029585798826020 ) ) ;
#22320=FACE_OUTER_BOUND ( 'NONE', #47205, .T. ) ;
#22334=ORIENTED_EDGE ( 'NONE', *, *, #62334, .F. ) ;
#22381=FACE_OUTER_BOUND ( 'NONE', #49056, .T. ) ;
#22439=CARTESIAN_POINT ( 'NONE',  ( -439.4229916354184979, 395.0000000000064801, -128.9497041420121093 ) ) ;
#22477=DIRECTION ( 'NONE',  ( -1.000000000000000000, 0.000000000000000000, -0.000000000000000000 ) ) ;
#22483=FACE_OUTER_BOUND ( 'NONE', #12240, .T. ) ;
#22508=EDGE_LOOP ( 'NONE', ( #55303, #59306, #20598, #49939 ) ) ;
#22514=CARTESIAN_POINT ( 'NONE',  ( 447.3372781065085633, 400.0000000000000568, -146.4497041420118251 ) ) ;
#22558=CARTESIAN_POINT ( 'NONE',  ( -443.1884682831975510, 394.9771332441898721, 92.74116978071172923 ) ) ;
#22584=DIRECTION ( 'NONE',  ( 1.387778780781445922E-16, -1.000000000000000000, -1.232595164407830946E-32 ) ) ;
#22611=FACE_OUTER_BOUND ( 'NONE', #12705, .T. ) ;
#22648=CARTESIAN_POINT ( 'NONE',  ( 442.3372781065085633, 369.9999999999999432, -141.4497041420118251 ) ) ;
#22656=CARTESIAN_POINT ( 'NONE',  ( 112.3013380801407521, 388.0000000000077307, 96.05029585798746439 ) ) ;
#22665=VECTOR ( 'NONE', #65262, 1000.000000000000000 ) ;
#22674=EDGE_LOOP ( 'NONE', ( #64873, #65635, #17115, #38266 ) ) ;
#22676=CLOSED_SHELL ( 'NONE', ( #15436, #27058, #28984, #13852, #3753, #3151, #49477, #30584, #69129, #30111, #38824, #31453, #62504, #15634, #10233 ) ) ;
#22681=VERTEX_POINT ( 'NONE', #35302 ) ;
#22684=CARTESIAN_POINT ( 'NONE',  ( -447.6627218934914367, 399.9999999999998863, -116.4497041420118393 ) ) ;
#22718=AXIS2_PLACEMENT_3D ( 'NONE', #47042, #30525, #57944 ) ;
#22730=CARTESIAN_POINT ( 'NONE',  ( 433.3728120124415568, 388.0000000000065938, 99.58582976392126795 ) ) ;
#22741=ORIENTED_EDGE ( 'NONE', *, *, #22961, .F. ) ;
#22756=DIRECTION ( 'NONE',  ( 0.000000000000000000, 0.000000000000000000, -1.000000000000000000 ) ) ;
#22785=VERTEX_POINT ( 'NONE', #38402 ) ;
#22795=EDGE_CURVE ( 'NONE', #34219, #60980, #1126, .T. ) ;
#22796=CARTESIAN_POINT ( 'NONE',  ( -452.6627218934914367, 399.9999999999998863, -111.4497041420118251 ) ) ;
#22804=VERTEX_POINT ( 'NONE', #33138 ) ;
#22806=VERTEX_POINT ( 'NONE', #54211 ) ;
#22845=CARTESIAN_POINT ( 'NONE',  ( -435.1627218934888788, 400.0000000000064801, -128.9497041420092387 ) ) ;
#22855=ORIENTED_EDGE ( 'NONE', *, *, #7337, .T. ) ;
#22864=ORIENTED_EDGE ( 'NONE', *, *, #2884, .T. ) ;
#22879=EDGE_CURVE ( 'NONE', #65265, #24702, #25371, .T. ) ;
#22910=CARTESIAN_POINT ( 'NONE',  ( -443.6229740799759043, 394.9118408295729523, 93.31364146883153410 ) ) ;
#22933=VERTEX_POINT ( 'NONE', #40489 ) ;
#22938=DIRECTION ( 'NONE',  ( 1.000000000000000000, 1.387778780781445922E-16, 0.000000000000000000 ) ) ;
#22943=EDGE_CURVE ( 'NONE', #59656, #46924, #3904, .T. ) ;
#22961=EDGE_CURVE ( 'NONE', #20867, #26715, #30293, .T. ) ;
#22991=DIRECTION ( 'NONE',  ( -1.000000000000000000, -1.110223024625118675E-14, 1.110223024625118675E-14 ) ) ;
#22995=VERTEX_POINT ( 'NONE', #62296 ) ;
#23001=CARTESIAN_POINT ( 'NONE',  ( 437.3372781065085633, 395.0000000000001137, -123.9497041420121235 ) ) ;
#23005=ORIENTED_EDGE ( 'NONE', *, *, #17153, .F. ) ;
#23006=VERTEX_POINT ( 'NONE', #51742 ) ;
#23012=VECTOR ( 'NONE', #43695, 1000.000000000000000 ) ;
#23073=VECTOR ( 'NONE', #58513, 1000.000000000000000 ) ;
#23080=DIRECTION ( 'NONE',  ( 0.000000000000000000, 1.000000000000000000, 0.000000000000000000 ) ) ;
#23082=VERTEX_POINT ( 'NONE', #46807 ) ;
#23103=DIRECTION ( 'NONE',  ( 0.7071067811865543451, 7.105427357601001070E-15, 0.7071067811865408004 ) ) ;
#23104=CARTESIAN_POINT ( 'NONE',  ( -439.4229916354185548, 388.0000000000064801, -133.9497041420121377 ) ) ;
#23111=DIRECTION ( 'NONE',  ( 1.000000000000000000, -3.344045254895050726E-17, 0.000000000000000000 ) ) ;
#23114=VECTOR ( 'NONE', #65998, 1000.000000000000000 ) ;
#23118=EDGE_CURVE ( 'NONE', #41002, #63860, #47597, .T. ) ;
#23122=CARTESIAN_POINT ( 'NONE',  ( 447.3372781065086201, 0.000000000000000000, 113.5502958579881749 ) ) ;
#23146=CARTESIAN_POINT ( 'NONE',  ( 447.3372781065085064, 400.0000000000001137, -146.4497041420118535 ) ) ;
#23151=LINE ( 'NONE', #22796, #48488 ) ;
#23167=AXIS2_PLACEMENT_3D ( 'NONE', #56792, #49752, #2985 ) ;
#23184=LINE ( 'NONE', #61833, #1521 ) ;
#23189=FACE_OUTER_BOUND ( 'NONE', #34610, .T. ) ;
#23197=LINE ( 'NONE', #19288, #20702 ) ;
#23201=LINE ( 'NONE', #67170, #7359 ) ;
#23209=FACE_OUTER_BOUND ( 'NONE', #4271, .T. ) ;
#23257=DIRECTION ( 'NONE',  ( 1.000000000000000000, 1.387778780781445922E-16, 0.000000000000000000 ) ) ;
#23355=EDGE_CURVE ( 'NONE', #63883, #11940, #24055, .T. ) ;
#23385=LINE ( 'NONE', #3298, #62677 ) ;
#23410=EDGE_LOOP ( 'NONE', ( #13990, #43564, #28892, #17082 ) ) ;
#23411=DIRECTION ( 'NONE',  ( 1.850371928290090422E-16, -1.000000000000000000, -1.110223024625156294E-16 ) ) ;
#23413=CARTESIAN_POINT ( 'NONE',  ( 447.3372781065085633, 399.9999999999998863, 113.5502958579881891 ) ) ;
#23427=MECHANICAL_DESIGN_GEOMETRIC_PRESENTATION_REPRESENTATION('',(#52623),#33570);
#23445=LINE ( 'NONE', #49795, #12676 ) ;
#23465=ORIENTED_EDGE ( 'NONE', *, *, #25816, .T. ) ;
#23466=CARTESIAN_POINT ( 'NONE',  ( 442.3372781065085633, 400.0000000000000568, -116.4497041420118393 ) ) ;
#23473=VERTEX_POINT ( 'NONE', #37805 ) ;
#23507=EDGE_CURVE ( 'NONE', #42064, #33355, #29697, .T. ) ;
#23511=FACE_OUTER_BOUND ( 'NONE', #65732, .T. ) ;
#23515=ORIENTED_EDGE ( 'NONE', *, *, #8681, .F. ) ;
#23528=SURFACE_STYLE_USAGE ( .BOTH. , #29147 ) ;
#23536=VECTOR ( 'NONE', #40025, 1000.000000000000000 ) ;
#23547=LINE ( 'NONE', #55896, #65653 ) ;
#23558=CARTESIAN_POINT ( 'NONE',  ( -452.6627218934914367, 399.9999999999998863, -146.4497041420118251 ) ) ;
#23565=DIRECTION ( 'NONE',  ( 0.000000000000000000, 0.000000000000000000, 1.000000000000000000 ) ) ;
#23569=DIRECTION ( 'NONE',  ( 0.000000000000000000, 3.469446951953616038E-17, -1.000000000000000000 ) ) ;
#23596=LINE ( 'NONE', #18309, #13004 ) ;
#23615=EDGE_CURVE ( 'NONE', #54414, #59656, #23547, .T. ) ;
#23631=DIRECTION ( 'NONE',  ( 1.110223024625155594E-14, 0.000000000000000000, 1.000000000000000000 ) ) ;
#23644=DIRECTION ( 'NONE',  ( -1.110223024625118675E-14, 0.000000000000000000, -1.000000000000000000 ) ) ;
#23655=ORIENTED_EDGE ( 'NONE', *, *, #35496, .F. ) ;
#23663=CARTESIAN_POINT ( 'NONE',  ( 437.3372781065085633, 399.9999999999998863, 108.5502958579881891 ) ) ;
#23676=ORIENTED_EDGE ( 'NONE', *, *, #52723, .T. ) ;
#23687=CARTESIAN_POINT ( 'NONE',  ( 447.3372781065086201, 0.000000000000000000, 78.55029585798817493 ) ) ;
#23710=VECTOR ( 'NONE', #59741, 1000.000000000000000 ) ;
#23735=EDGE_CURVE ( 'NONE', #48439, #4870, #23197, .T. ) ;
#23736=CARTESIAN_POINT ( 'NONE',  ( -447.6627218934912662, 369.9999999999998295, 108.5502958579877060 ) ) ;
#23739=ORIENTED_EDGE ( 'NONE', *, *, #3644, .F. ) ;
#23757=B_SPLINE_CURVE_WITH_KNOTS ( 'NONE', 3,
 ( #10926, #64053, #48538, #49246, #59803, #69333, #38715, #38358, #11270, #65098 ),
 .UNSPECIFIED., .F., .F.,
 ( 4, 2, 2, 2, 4 ),
 ( 0.004323147273503904695, 0.005401969756752490054, 0.006480792240001076281, 0.007559614723249662507, 0.008638437206498247867 ),
 .UNSPECIFIED. ) ;
#23758=LINE ( 'NONE', #51186, #6857 ) ;
#23760=CARTESIAN_POINT ( 'NONE',  ( 412.3372781065089612, 397.0710678118719557, -111.4497041420121803 ) ) ;
#23778=DIRECTION ( 'NONE',  ( 1.387778780781445429E-16, -1.000000000000000000, -3.081487911019577365E-33 ) ) ;
#23779=DIRECTION ( 'NONE',  ( 9.899279560275165216E-15, -1.665334536937735057E-16, 1.000000000000000000 ) ) ;
#23791=CARTESIAN_POINT ( 'NONE',  ( -440.1146514826274938, 400.0000000000065370, -133.9016337311479958 ) ) ;
#23819=EDGE_LOOP ( 'NONE', ( #28770, #59880, #41561, #23465, #46500, #57788, #55468, #3716, #5513, #10648, #57007, #51608, #43189, #35925, #15070 ) ) ;
#23829=LINE ( 'NONE', #18546, #52561 ) ;
#23850=CLOSED_SHELL ( 'NONE', ( #67763, #61553, #64908, #48239, #40342, #69561, #14145, #50110, #28282 ) ) ;
#23856=LINE ( 'NONE', #18570, #23536 ) ;
#23870=ORIENTED_EDGE ( 'NONE', *, *, #65109, .T. ) ;
#23921=ORIENTED_EDGE ( 'NONE', *, *, #3257, .T. ) ;
#23931=CARTESIAN_POINT ( 'NONE',  ( 429.8372781065084496, 400.0000000000042633, 96.05029585798401115 ) ) ;
#23949=CARTESIAN_POINT ( 'NONE',  ( -422.6627218934906978, 394.9999999999998295, 83.55029585798750702 ) ) ;
#23958=CARTESIAN_POINT ( 'NONE',  ( -447.6627218934914367, 399.9999999999998863, -136.4497041420118251 ) ) ;
#23966=PLANE ( 'NONE',  #59139 ) ;
#23968=EDGE_CURVE ( 'NONE', #46238, #35076, #55452, .T. ) ;
#23975=CARTESIAN_POINT ( 'NONE',  ( 442.3372781065085633, 370.0000000000038085, 108.5502958579885870 ) ) ;
#23989=DIRECTION ( 'NONE',  ( -1.001915251000354105E-14, 1.000000000000000000, -5.551115123125782702E-17 ) ) ;
#24010=CARTESIAN_POINT ( 'NONE',  ( 447.3372781065086770, 400.0000000000000568, -146.4497041420117966 ) ) ;
#24024=EDGE_LOOP ( 'NONE', ( #68728, #56549, #46570, #8401 ) ) ;
#24029=DIRECTION ( 'NONE',  ( -1.850371928290090422E-16, 1.000000000000000000, 1.110223024625156171E-16 ) ) ;
#24049=LINE ( 'NONE', #25445, #3490 ) ;
#24055=( BOUNDED_CURVE ( )  B_SPLINE_CURVE ( 3, ( #46283, #15320, #52598, #51914 ),
 .UNSPECIFIED., .F., .F. ) 
 B_SPLINE_CURVE_WITH_KNOTS ( ( 4, 4 ),
 ( 0.000000000000000000, 1.570796326794796638 ),
 .UNSPECIFIED. ) 
 CURVE ( )  GEOMETRIC_REPRESENTATION_ITEM ( )  RATIONAL_B_SPLINE_CURVE ( ( 1.000000000000000000, 0.8047378541243885852, 0.8047378541243885852, 1.000000000000000000 ) ) 
 REPRESENTATION_ITEM ( '' )  );
#24059=DIRECTION ( 'NONE',  ( -1.020422603260505347E-14, 1.000000000000000000, 5.551115123125782702E-17 ) ) ;
#24061=UNCERTAINTY_MEASURE_WITH_UNIT (LENGTH_MEASURE( 1.000000000000000082E-05 ), #31232, 'distance_accuracy_value', 'NONE');
#24076=FACE_OUTER_BOUND ( 'NONE', #39827, .T. ) ;
#24077=ADVANCED_FACE ( 'NONE', ( #10370 ), #59250, .T. ) ;
#24079=AXIS2_PLACEMENT_3D ( 'NONE', #67744, #57873, #52587 ) ;
#24102=ADVANCED_FACE ( 'NONE', ( #22320 ), #20936, .T. ) ;
#24107=ADVANCED_FACE ( 'NONE', ( #64890 ), #11759, .F. ) ;
#24113=CARTESIAN_POINT ( 'NONE',  ( 442.3372781065085633, 370.0000000000001137, -141.4497041420118251 ) ) ;
#24124=VECTOR ( 'NONE', #54003, 1000.000000000000000 ) ;
#24192=CIRCLE ( 'NONE', #19658, 5.000000000000087930 ) ;
#24196=AXIS2_PLACEMENT_3D ( 'NONE', #14626, #41369, #67412 ) ;
#24200=DIRECTION ( 'NONE',  ( -2.921639538487254261E-16, -1.134144525784205431E-35, -1.000000000000000000 ) ) ;
#24241=VERTEX_POINT ( 'NONE', #29684 ) ;
#24243=CARTESIAN_POINT ( 'NONE',  ( -452.6627218934859798, 400.0000000000064801, -146.4497041420121377 ) ) ;
#24252=EDGE_CURVE ( 'NONE', #12094, #50931, #41622, .T. ) ;
#24290=CARTESIAN_POINT ( 'NONE',  ( -450.6627218934913230, 217.8591479523843475, -111.4497041420117966 ) ) ;
#24303=CARTESIAN_POINT ( 'NONE',  ( -430.1627218934915504, 394.9999999999998295, -123.9497041420119530 ) ) ;
#24336=VERTEX_POINT ( 'NONE', #42981 ) ;
#24345=ORIENTED_EDGE ( 'NONE', *, *, #2568, .F. ) ;
#24346=CARTESIAN_POINT ( 'NONE',  ( 442.3372781065086201, 395.0000000000043201, 108.5502958579839117 ) ) ;
#24353=LINE ( 'NONE', #3240, #33711 ) ;
#24367=EDGE_CURVE ( 'NONE', #29979, #58622, #42313, .T. ) ;
#24393=CARTESIAN_POINT ( 'NONE',  ( -450.6627218934913230, 177.8591479523843475, 78.55029585798814651 ) ) ;
#24410=FACE_OUTER_BOUND ( 'NONE', #62347, .T. ) ;
#24412=ADVANCED_FACE ( 'NONE', ( #15235 ), #47570, .F. ) ;
#24438=AXIS2_PLACEMENT_3D ( 'NONE', #1787, #60514, #7046 ) ;
#24473=( BOUNDED_CURVE ( )  B_SPLINE_CURVE ( 3, ( #20857, #26486, #52849, #63430 ),
 .UNSPECIFIED., .F., .F. ) 
 B_SPLINE_CURVE_WITH_KNOTS ( ( 4, 4 ),
 ( 1.570796326794897224, 3.141592653589780237 ),
 .UNSPECIFIED. ) 
 CURVE ( )  GEOMETRIC_REPRESENTATION_ITEM ( )  RATIONAL_B_SPLINE_CURVE ( ( 1.000000000000000000, 0.8047378541243681571, 0.8047378541243681571, 1.000000000000000000 ) ) 
 REPRESENTATION_ITEM ( '' )  );
#24475=VECTOR ( 'NONE', #49462, 1000.000000000000000 ) ;
#24479=ORIENTED_EDGE ( 'NONE', *, *, #3959, .T. ) ;
#24489=CARTESIAN_POINT ( 'NONE',  ( -452.6627218934913230, 399.9999999999997726, 113.5502958579881891 ) ) ;
#24527=VERTEX_POINT ( 'NONE', #66562 ) ;
#24529=DIRECTION ( 'NONE',  ( 1.000000000000000000, 0.000000000000000000, 0.000000000000000000 ) ) ;
#24537=VECTOR ( 'NONE', #5412, 1000.000000000000000 ) ;
#24539=LINE ( 'NONE', #35778, #60058 ) ;
#24543=ORIENTED_EDGE ( 'NONE', *, *, #22961, .T. ) ;
#24544=AXIS2_PLACEMENT_3D ( 'NONE', #4319, #14860, #30358 ) ;
#24554=EDGE_CURVE ( 'NONE', #17392, #22806, #31251, .T. ) ;
#24562=ORIENTED_EDGE ( 'NONE', *, *, #65039, .F. ) ;
#24572=ORIENTED_EDGE ( 'NONE', *, *, #12077, .F. ) ;
#24594=ADVANCED_FACE ( 'NONE', ( #43855 ), #48773, .T. ) ;
#24610=CYLINDRICAL_SURFACE ( 'NONE', #66111, 5.000000000000004441 ) ;
#24625=VECTOR ( 'NONE', #12407, 1000.000000000000000 ) ;
#24656=CARTESIAN_POINT ( 'NONE',  ( 447.3372781065086201, 0.000000000000000000, 78.55029585798817493 ) ) ;
#24661=DIRECTION ( 'NONE',  ( 1.000000000000000000, 0.000000000000000000, 0.000000000000000000 ) ) ;
#24687=ORIENTED_EDGE ( 'NONE', *, *, #23507, .F. ) ;
#24699=ADVANCED_FACE ( 'NONE', ( #29431 ), #3057, .F. ) ;
#24700=EDGE_LOOP ( 'NONE', ( #30321, #1391, #38693, #37024 ) ) ;
#24701=CARTESIAN_POINT ( 'NONE',  ( -440.1146514826278917, 394.9999999999955094, 101.0022254471289358 ) ) ;
#24702=VERTEX_POINT ( 'NONE', #34380 ) ;
#24721=CARTESIAN_POINT ( 'NONE',  ( -442.6627218934912662, 394.9999999999998295, 113.5502958579882034 ) ) ;
#24737=ORIENTED_EDGE ( 'NONE', *, *, #24367, .F. ) ;
#24747=CARTESIAN_POINT ( 'NONE',  ( -417.6627218934913230, 219.4906275429376308, -144.4497041420118819 ) ) ;
#24757=DIRECTION ( 'NONE',  ( -0.000000000000000000, -6.405132834375902056E-16, 1.000000000000000000 ) ) ;
#24804=VECTOR ( 'NONE', #1640, 1000.000000000000000 ) ;
#24806=EDGE_LOOP ( 'NONE', ( #27339, #26415, #57735, #51065 ) ) ;
#24821=FACE_OUTER_BOUND ( 'NONE', #14937, .T. ) ;
#24822=CARTESIAN_POINT ( 'NONE',  ( 412.3372781065083927, 397.0710678118695114, 78.55029585798419589 ) ) ;
#24838=EDGE_CURVE ( 'NONE', #16988, #41527, #46989, .T. ) ;
#24880=EDGE_CURVE ( 'NONE', #20962, #8527, #42147, .T. ) ;
#24903=CARTESIAN_POINT ( 'NONE',  ( 412.3372781065085633, 219.4906275429376308, -144.4497041420117682 ) ) ;
#24917=CARTESIAN_POINT ( 'NONE',  ( -447.6627218934919483, 370.0000000000056275, -141.4497041420121661 ) ) ;
#24935=ORIENTED_EDGE ( 'NONE', *, *, #58344, .T. ) ;
#24967=DIRECTION ( 'NONE',  ( -1.000000000000000000, -1.001918046209079887E-14, 9.729495617646301779E-15 ) ) ;
#25001=ORIENTED_EDGE ( 'NONE', *, *, #26286, .T. ) ;
#25023=LINE ( 'NONE', #23975, #6436 ) ;
#25036=AXIS2_PLACEMENT_3D ( 'NONE', #29613, #46136, #34573 ) ;
#25057=DIRECTION ( 'NONE',  ( 0.7071067811865475727, 5.551115123125781470E-17, -0.7071067811865474617 ) ) ;
#25070=DIRECTION ( 'NONE',  ( -9.109522253334599209E-16, -1.000000000000000000, 0.000000000000000000 ) ) ;
#25106=VECTOR ( 'NONE', #32595, 1000.000000000000000 ) ;
#25107=PLANE ( 'NONE',  #12684 ) ;
#25115=LINE ( 'NONE', #9621, #14934 ) ;
#25141=STYLED_ITEM ( 'NONE', ( #56926 ), #40015 ) ;
#25200=VECTOR ( 'NONE', #31324, 1000.000000000000000 ) ;
#25246=DIRECTION ( 'NONE',  ( 4.314083075427411048E-32, 1.000000000000000000, 6.123233995736763571E-17 ) ) ;
#25253=DIRECTION ( 'NONE',  ( -1.000000000000000000, -1.110223024625155594E-14, 1.110223024625155594E-14 ) ) ;
#25257=EDGE_CURVE ( 'NONE', #29332, #27359, #3651, .T. ) ;
#25295=DIRECTION ( 'NONE',  ( 9.115745035929406798E-64, -3.469446951953612956E-17, 1.000000000000000000 ) ) ;
#25333=DIRECTION ( 'NONE',  ( 0.000000000000000000, -1.000000000000000000, 0.000000000000000000 ) ) ;
#25337=ORIENTED_EDGE ( 'NONE', *, *, #45618, .T. ) ;
#25362=ORIENTED_EDGE ( 'NONE', *, *, #61391, .F. ) ;
#25370=CARTESIAN_POINT ( 'NONE',  ( -417.6627218934913230, 399.9999999999998295, 113.5502958579882602 ) ) ;
#25371=LINE ( 'NONE', #13081, #10550 ) ;
#25372=VERTEX_POINT ( 'NONE', #43343 ) ;
#25380=DIRECTION ( 'NONE',  ( 9.109522253334613014E-16, 1.000000000000000000, -3.889846672687432470E-31 ) ) ;
#25421=CARTESIAN_POINT ( 'NONE',  ( 447.3372781065086201, 0.000000000000000000, -116.4497041420118393 ) ) ;
#25431=VECTOR ( 'NONE', #51457, 1000.000000000000000 ) ;
#25445=CARTESIAN_POINT ( 'NONE',  ( 2.337278106504167230, 395.0000000000000000, -341.4497041420117966 ) ) ;
#25472=CARTESIAN_POINT ( 'NONE',  ( -417.6627218934917778, 400.0000000000064801, -111.4497041420121661 ) ) ;
#25524=DIRECTION ( 'NONE',  ( -1.020422603260505347E-14, 1.000000000000000000, 5.551115123125782702E-17 ) ) ;
#25527=ORIENTED_EDGE ( 'NONE', *, *, #69155, .T. ) ;
#25559=ORIENTED_EDGE ( 'NONE', *, *, #50885, .F. ) ;
#25596=CARTESIAN_POINT ( 'NONE',  ( -452.6627218934913230, 399.9999999999997726, 83.55029585798818914 ) ) ;
#25614=SURFACE_STYLE_USAGE ( .BOTH. , #15045 ) ;
#25620=CARTESIAN_POINT ( 'NONE',  ( -447.6627218934913799, 369.9999999999998295, -141.4497041420117966 ) ) ;
#25635=VECTOR ( 'NONE', #41114, 1000.000000000000000 ) ;
#25643=EDGE_LOOP ( 'NONE', ( #43314, #13413, #2335, #37991 ) ) ;
#25665=ORIENTED_EDGE ( 'NONE', *, *, #62080, .T. ) ;
#25671=DIRECTION ( 'NONE',  ( 1.000000000000000000, 1.019401483866766449E-14, -9.729483335668566592E-15 ) ) ;
#25695=ORIENTED_EDGE ( 'NONE', *, *, #5545, .F. ) ;
#25696=DIRECTION ( 'NONE',  ( -1.000000000000000000, -0.000000000000000000, -0.000000000000000000 ) ) ;
#25724=ORIENTED_EDGE ( 'NONE', *, *, #51957, .F. ) ;
#25784=DIRECTION ( 'NONE',  ( -0.7071067811865476838, 6.441404958702661839E-16, -0.7071067811865474617 ) ) ;
#25785=AXIS2_PLACEMENT_3D ( 'NONE', #14560, #2979, #2622 ) ;
#25816=EDGE_CURVE ( 'NONE', #57474, #46683, #16878, .T. ) ;
#25835=CARTESIAN_POINT ( 'NONE',  ( -452.6627218934913230, 217.8591479523843475, -111.4497041420117966 ) ) ;
#25848=LINE ( 'NONE', #47963, #24537 ) ;
#25865=PLANE ( 'NONE',  #52791 ) ;
#25870=FILL_AREA_STYLE ('',( #15308 ) ) ;
#25880=CARTESIAN_POINT ( 'NONE',  ( 112.3013380801408800, 395.0000000000065938, -133.9497041420121377 ) ) ;
#25882=DIRECTION ( 'NONE',  ( 1.850169831522831466E-16, -1.000000000000000000, 5.551115123125781470E-17 ) ) ;
#25913=CARTESIAN_POINT ( 'NONE',  ( 447.3372781065086201, 400.0000000000044338, 113.5502958579838122 ) ) ;
#25936=AXIS2_PLACEMENT_3D ( 'NONE', #34116, #13356, #60833 ) ;
#25949=SURFACE_STYLE_FILL_AREA ( #57266 ) ;
#25952=CARTESIAN_POINT ( 'NONE',  ( 447.3372781065086201, 0.000000000000000000, -116.4497041420118393 ) ) ;
#25953=LINE ( 'NONE', #52667, #3547 ) ;
#25954=FACE_OUTER_BOUND ( 'NONE', #27294, .T. ) ;
#25971=EDGE_CURVE ( 'NONE', #9014, #22785, #68123, .T. ) ;
#25973=FACE_OUTER_BOUND ( 'NONE', #53635, .T. ) ;
#25994=CIRCLE ( 'NONE', #64136, 5.000000000000004441 ) ;
#26005=MECHANICAL_DESIGN_GEOMETRIC_PRESENTATION_REPRESENTATION('',(#33887),#30515);
#26014=LINE ( 'NONE', #4214, #21501 ) ;
#26015=ORIENTED_EDGE ( 'NONE', *, *, #33592, .F. ) ;
#26026=EDGE_LOOP ( 'NONE', ( #27056, #21125, #21992, #4159 ) ) ;
#26054=ORIENTED_EDGE ( 'NONE', *, *, #58344, .F. ) ;
#26059=SURFACE_STYLE_USAGE ( .BOTH. , #41541 ) ;
#26091=AXIS2_PLACEMENT_3D ( 'NONE', #25913, #52290, #4450 ) ;
#26115=DIRECTION ( 'NONE',  ( -1.000000000000000000, -1.001918046209079887E-14, 9.729495617646301779E-15 ) ) ;
#26174=ORIENTED_EDGE ( 'NONE', *, *, #1352, .T. ) ;
#26178=VECTOR ( 'NONE', #23778, 1000.000000000000000 ) ;
#26188=EDGE_CURVE ( 'NONE', #8527, #68125, #53559, .T. ) ;
#26217=DIRECTION ( 'NONE',  ( 1.000000000000000000, 1.387778780781445922E-16, 0.000000000000000000 ) ) ;
#26220=CARTESIAN_POINT ( 'NONE',  ( -422.6627218934913230, 399.9999999999997726, 113.5502958579881891 ) ) ;
#26233=ORIENTED_EDGE ( 'NONE', *, *, #48709, .F. ) ;
#26237=AXIS2_PLACEMENT_3D ( 'NONE', #53077, #41860, #4564 ) ;
#26246=CARTESIAN_POINT ( 'NONE',  ( 447.3372781065085633, 400.0000000000000568, -116.4497041420118393 ) ) ;
#26251=DIRECTION ( 'NONE',  ( 1.387778780781445922E-16, -1.000000000000000000, -1.232595164407830946E-32 ) ) ;
#26271=CARTESIAN_POINT ( 'NONE',  ( -417.6627218934913230, 399.9999999999997726, 113.5502958579881891 ) ) ;
#26283=VECTOR ( 'NONE', #6909, 1000.000000000000000 ) ;
#26286=EDGE_CURVE ( 'NONE', #21328, #23006, #53899, .T. ) ;
#26298=DIRECTION ( 'NONE',  ( -1.110223024625155594E-14, 0.000000000000000000, -1.000000000000000000 ) ) ;
#26309=( NAMED_UNIT ( * ) PLANE_ANGLE_UNIT ( ) SI_UNIT ( $, .RADIAN. ) );
#26324=EDGE_CURVE ( 'NONE', #15602, #68802, #807, .T. ) ;
#26344=DIRECTION ( 'NONE',  ( -1.000000000000000000, -1.387778780781445922E-16, 0.000000000000000000 ) ) ;
#26351=EDGE_CURVE ( 'NONE', #6937, #910, #17323, .T. ) ;
#26352=ADVANCED_FACE ( 'NONE', ( #15942 ), #13450, .T. ) ;
#26368=CYLINDRICAL_SURFACE ( 'NONE', #11406, 5.000000000000004441 ) ;
#26400=VERTEX_POINT ( 'NONE', #67281 ) ;
#26415=ORIENTED_EDGE ( 'NONE', *, *, #19611, .T. ) ;
#26416=FACE_OUTER_BOUND ( 'NONE', #3044, .T. ) ;
#26484=CARTESIAN_POINT ( 'NONE',  ( 429.8372781065087906, 388.0000000000066507, -128.9497041420121093 ) ) ;
#26485=DIRECTION ( 'NONE',  ( 0.7071067811865473507, 0.000000000000000000, -0.7071067811865477948 ) ) ;
#26486=CARTESIAN_POINT ( 'NONE',  ( -419.7337897053570828, 394.9999999999957367, 80.62136366985768632 ) ) ;
#26512=EDGE_CURVE ( 'NONE', #16392, #29739, #41904, .T. ) ;
#26513=VECTOR ( 'NONE', #67553, 1000.000000000000000 ) ;
#26519=CARTESIAN_POINT ( 'NONE',  ( 112.3013380801407379, 395.0000000000010800, 101.0502958579874644 ) ) ;
#26527=LINE ( 'NONE', #16993, #32262 ) ;
#26584=ORIENTED_EDGE ( 'NONE', *, *, #67580, .F. ) ;
#26612=DIRECTION ( 'NONE',  ( -1.000000000000000000, -1.001918046209079887E-14, 9.729495617646301779E-15 ) ) ;
#26615=EDGE_LOOP ( 'NONE', ( #66360, #17795, #45988, #44079 ) ) ;
#26660=ORIENTED_EDGE ( 'NONE', *, *, #2953, .T. ) ;
#26700=ORIENTED_EDGE ( 'NONE', *, *, #46307, .F. ) ;
#26704=DIRECTION ( 'NONE',  ( -1.020422603260505347E-14, 1.000000000000000000, 5.551115123125782702E-17 ) ) ;
#26715=VERTEX_POINT ( 'NONE', #30683 ) ;
#26723=CARTESIAN_POINT ( 'NONE',  ( 442.3372781065081654, 367.0710678118697388, 108.5502958579838975 ) ) ;
#26724=PLANE ( 'NONE',  #1849 ) ;
#26727=DIRECTION ( 'NONE',  ( 9.740878893424455404E-21, -6.106226635438359986E-16, 1.000000000000000000 ) ) ;
#26755=CARTESIAN_POINT ( 'NONE',  ( 424.8372781065089043, 395.0000000000065938, -123.9497041420121235 ) ) ;
#26762=LINE ( 'NONE', #723, #12671 ) ;
#26763=ORIENTED_EDGE ( 'NONE', *, *, #10304, .F. ) ;
#26819=STYLED_ITEM ( 'NONE', ( #50586 ), #64175 ) ;
#26840=DIRECTION ( 'NONE',  ( 0.000000000000000000, 0.000000000000000000, 1.000000000000000000 ) ) ;
#26868=CARTESIAN_POINT ( 'NONE',  ( 447.3372781065086201, 0.000000000000000000, -111.4497041420118251 ) ) ;
#26872=DIRECTION ( 'NONE',  ( -1.110223024625156294E-16, 0.000000000000000000, 1.000000000000000000 ) ) ;
#26877=ORIENTED_EDGE ( 'NONE', *, *, #44619, .T. ) ;
#26923=ADVANCED_FACE ( 'NONE', ( #51714 ), #2833, .T. ) ;
#26942=LINE ( 'NONE', #17065, #16210 ) ;
#26944=VERTEX_POINT ( 'NONE', #2147 ) ;
#26958=CIRCLE ( 'NONE', #6733, 5.000000000000004441 ) ;
#26962=DIRECTION ( 'NONE',  ( -1.000000000000000000, -1.387778780781445429E-16, 0.000000000000000000 ) ) ;
#27009=EDGE_CURVE ( 'NONE', #41527, #1580, #16825, .T. ) ;
#27017=CARTESIAN_POINT ( 'NONE',  ( 447.3372781065085633, 399.9999999999998863, 78.55029585798817493 ) ) ;
#27037=DIRECTION ( 'NONE',  ( -6.405132834375901070E-16, 1.000000000000000000, 6.405132834375902056E-16 ) ) ;
#27048=CARTESIAN_POINT ( 'NONE',  ( 417.3372781065085633, 395.0000000000000568, -116.4497041420117824 ) ) ;
#27056=ORIENTED_EDGE ( 'NONE', *, *, #3959, .F. ) ;
#27058=ADVANCED_FACE ( 'NONE', ( #37592 ), #65734, .T. ) ;
#27071=FACE_OUTER_BOUND ( 'NONE', #24700, .T. ) ;
#27126=( GEOMETRIC_REPRESENTATION_CONTEXT ( 3 ) GLOBAL_UNCERTAINTY_ASSIGNED_CONTEXT ( ( #38855 ) ) GLOBAL_UNIT_ASSIGNED_CONTEXT ( ( #27409, #21785, #37621 ) ) REPRESENTATION_CONTEXT ( 'NONE', 'WORKASPACE' ) );
#27130=ADVANCED_FACE ( 'NONE', ( #68085 ), #41343, .T. ) ;
#27180=LINE ( 'NONE', #60590, #24625 ) ;
#27197=ORIENTED_EDGE ( 'NONE', *, *, #7613, .F. ) ;
#27211=EDGE_CURVE ( 'NONE', #31046, #12220, #37424, .T. ) ;
#27234=DIRECTION ( 'NONE',  ( 1.850169831522831466E-16, -1.000000000000000000, 5.551115123125781470E-17 ) ) ;
#27239=DIRECTION ( 'NONE',  ( -1.000000000000000000, 0.000000000000000000, 0.000000000000000000 ) ) ;
#27250=DIRECTION ( 'NONE',  ( 5.551115123125781716E-16, -3.469446951953605561E-17, 1.000000000000000000 ) ) ;
#27261=FACE_OUTER_BOUND ( 'NONE', #33826, .T. ) ;
#27286=EDGE_CURVE ( 'NONE', #48080, #62663, #31471, .T. ) ;
#27294=EDGE_LOOP ( 'NONE', ( #47721, #19861, #48475, #40549 ) ) ;
#27310=( NAMED_UNIT ( * ) PLANE_ANGLE_UNIT ( ) SI_UNIT ( $, .RADIAN. ) );
#27323=VECTOR ( 'NONE', #18679, 1000.000000000000000 ) ;
#27326=CARTESIAN_POINT ( 'NONE',  ( 412.3372781065085633, 400.0000000000000568, -111.4497041420117682 ) ) ;
#27339=ORIENTED_EDGE ( 'NONE', *, *, #25816, .F. ) ;
#27340=DIRECTION ( 'NONE',  ( 1.001917982681609001E-14, -1.000000000000000000, -5.551115123125782702E-17 ) ) ;
#27341=PLANE ( 'NONE',  #10505 ) ;
#27357=( GEOMETRIC_REPRESENTATION_CONTEXT ( 3 ) GLOBAL_UNCERTAINTY_ASSIGNED_CONTEXT ( ( #1552 ) ) GLOBAL_UNIT_ASSIGNED_CONTEXT ( ( #45317, #2761, #13323 ) ) REPRESENTATION_CONTEXT ( 'NONE', 'WORKASPACE' ) );
#27359=VERTEX_POINT ( 'NONE', #22296 ) ;
#27366=EDGE_CURVE ( 'NONE', #14174, #4675, #6470, .T. ) ;
#27373=ORIENTED_EDGE ( 'NONE', *, *, #36201, .T. ) ;
#27386=DIRECTION ( 'NONE',  ( -1.387778780781445429E-16, 1.000000000000000000, 3.081487911019577365E-33 ) ) ;
#27409=( LENGTH_UNIT ( ) NAMED_UNIT ( * ) SI_UNIT ( .MILLI., .METRE. ) );
#27415=CARTESIAN_POINT ( 'NONE',  ( 447.3372781065085633, 370.0000000000001137, -146.4497041420116830 ) ) ;
#27422=AXIS2_PLACEMENT_3D ( 'NONE', #65402, #49544, #10531 ) ;
#27434=ORIENTED_EDGE ( 'NONE', *, *, #56725, .T. ) ;
#27444=DIRECTION ( 'NONE',  ( 1.000000000000000000, 1.387778780781443950E-16, 0.000000000000000000 ) ) ;
#27446=PLANE ( 'NONE',  #24438 ) ;
#27452=CARTESIAN_POINT ( 'NONE',  ( 417.3372781065085633, 394.9999999999999432, 83.55029585798834546 ) ) ;
#27468=VECTOR ( 'NONE', #34789, 1000.000000000000000 ) ;
#27478=FACE_OUTER_BOUND ( 'NONE', #11260, .T. ) ;
#27484=EDGE_CURVE ( 'NONE', #13320, #29891, #1776, .T. ) ;
#27504=LINE ( 'NONE', #56241, #18354 ) ;
#27509=ORIENTED_EDGE ( 'NONE', *, *, #15323, .F. ) ;
#27510=DIRECTION ( 'NONE',  ( -1.850371928290090422E-16, 1.000000000000000000, 1.110223024625156171E-16 ) ) ;
#27512=AXIS2_PLACEMENT_3D ( 'NONE', #40631, #62794, #4055 ) ;
#27514=DIRECTION ( 'NONE',  ( -0.000000000000000000, -6.405132834375902056E-16, 1.000000000000000000 ) ) ;
#27521=PLANE ( 'NONE',  #28230 ) ;
#27545=DIRECTION ( 'NONE',  ( 1.000000000000000000, 1.019401483866766449E-14, -9.729483335668566592E-15 ) ) ;
#27552=DIRECTION ( 'NONE',  ( 1.940875045995544638E-32, -1.110223024625156171E-16, 1.000000000000000000 ) ) ;
#27563=CARTESIAN_POINT ( 'NONE',  ( 442.3372781065086201, 0.000000000000000000, -116.4497041420118393 ) ) ;
#27585=CARTESIAN_POINT ( 'NONE',  ( 447.3372781065085633, 399.9999999999998863, 78.55029585798817493 ) ) ;
#27588=CARTESIAN_POINT ( 'NONE',  ( 424.8372781065089043, 400.0000000000067075, -123.9497041420121235 ) ) ;
#27609=EDGE_LOOP ( 'NONE', ( #4507, #5731, #9091, #31097, #3319 ) ) ;
#27617=LINE ( 'NONE', #23413, #54429 ) ;
#27673=DIRECTION ( 'NONE',  ( 1.387778780781445429E-16, -1.000000000000000000, -3.081487911019577365E-33 ) ) ;
#27691=CARTESIAN_POINT ( 'NONE',  ( -422.6627218934913799, 394.9999999999998295, -116.4497041420117824 ) ) ;
#27695=PLANE ( 'NONE',  #48130 ) ;
#27712=ORIENTED_EDGE ( 'NONE', *, *, #55999, .T. ) ;
#27739=DIRECTION ( 'NONE',  ( -0.7071067811865474617, -9.058225723175622340E-16, 0.7071067811865474617 ) ) ;
#27778=CARTESIAN_POINT ( 'NONE',  ( 50.98853755884136518, 400.0000000000071054, 96.05029585798814651 ) ) ;
#27785=ORIENTED_EDGE ( 'NONE', *, *, #23355, .F. ) ;
#27847=EDGE_LOOP ( 'NONE', ( #58208, #22037, #5806, #17721 ) ) ;
#27861=EDGE_CURVE ( 'NONE', #58622, #66845, #43263, .T. ) ;
#27891=EDGE_CURVE ( 'NONE', #51413, #37758, #11554, .T. ) ;
#27894=DIRECTION ( 'NONE',  ( -7.596454196607838998E-65, 3.469446951953615421E-17, -1.000000000000000000 ) ) ;
#27908=LINE ( 'NONE', #53235, #59198 ) ;
#27922=CIRCLE ( 'NONE', #49242, 5.000000000000004441 ) ;
#27930=CARTESIAN_POINT ( 'NONE',  ( 412.3372781065085633, 179.4906275429376024, 111.5502958579881749 ) ) ;
#27955=DIRECTION ( 'NONE',  ( -0.000000000000000000, -1.000000000000000000, -0.000000000000000000 ) ) ;
#27958=DIRECTION ( 'NONE',  ( -1.000000000000000000, -3.697785493223491743E-32, 0.000000000000000000 ) ) ;
#28010=EDGE_CURVE ( 'NONE', #45699, #38702, #59403, .T. ) ;
#28036=DIRECTION ( 'NONE',  ( 0.7071067811865475727, 0.000000000000000000, 0.7071067811865474617 ) ) ;
#28042=CARTESIAN_POINT ( 'NONE',  ( -442.6627218934912662, 394.9999999999998295, 113.5502958579882034 ) ) ;
#28050=VECTOR ( 'NONE', #69179, 1000.000000000000000 ) ;
#28056=ORIENTED_EDGE ( 'NONE', *, *, #65706, .F. ) ;
#28065=CARTESIAN_POINT ( 'NONE',  ( -430.1627218934918346, 399.9999999999952820, 91.05029585799256608 ) ) ;
#28079=CYLINDRICAL_SURFACE ( 'NONE', #3237, 5.000000000000004441 ) ;
#28090=ORIENTED_EDGE ( 'NONE', *, *, #5952, .T. ) ;
#28103=ORIENTED_EDGE ( 'NONE', *, *, #22795, .F. ) ;
#28106=VERTEX_POINT ( 'NONE', #17901 ) ;
#28115=VECTOR ( 'NONE', #45195, 1000.000000000000000 ) ;
#28119=FACE_OUTER_BOUND ( 'NONE', #29051, .T. ) ;
#28132=CARTESIAN_POINT ( 'NONE',  ( 447.3372781065085633, 399.9999999999998863, 78.55029585798817493 ) ) ;
#28141=LINE ( 'NONE', #16550, #9504 ) ;
#28172=EDGE_CURVE ( 'NONE', #54414, #46955, #19948, .T. ) ;
#28217=ORIENTED_EDGE ( 'NONE', *, *, #64221, .F. ) ;
#28230=AXIS2_PLACEMENT_3D ( 'NONE', #65523, #48963, #803 ) ;
#28252=EDGE_CURVE ( 'NONE', #46731, #34711, #45606, .T. ) ;
#28273=CYLINDRICAL_SURFACE ( 'NONE', #31164, 5.000000000000004441 ) ;
#28276=EDGE_CURVE ( 'NONE', #25372, #40455, #57953, .T. ) ;
#28279=CARTESIAN_POINT ( 'NONE',  ( -447.6627218934915504, 392.9289321881299770, 108.5502958579924950 ) ) ;
#28280=ADVANCED_FACE ( 'NONE', ( #21018 ), #41437, .T. ) ;
#28282=ADVANCED_FACE ( 'NONE', ( #20662 ), #42121, .T. ) ;
#28296=VERTEX_POINT ( 'NONE', #35819 ) ;
#28297=DIRECTION ( 'NONE',  ( 0.7071067811865405783, 7.105427357601001070E-15, -0.7071067811865545671 ) ) ;
#28334=DIRECTION ( 'NONE',  ( 1.387778780781445922E-16, -1.000000000000000000, -1.232595164407830946E-32 ) ) ;
#28361=LINE ( 'NONE', #39277, #26283 ) ;
#28370=DIRECTION ( 'NONE',  ( 1.343643437439745986E-14, 1.000000000000000000, 1.110223024625156171E-16 ) ) ;
#28378=DIRECTION ( 'NONE',  ( -6.405132834375901070E-16, 1.000000000000000000, 6.405132834375902056E-16 ) ) ;
#28396=VERTEX_POINT ( 'NONE', #5857 ) ;
#28405=ORIENTED_EDGE ( 'NONE', *, *, #43655, .F. ) ;
#28450=CARTESIAN_POINT ( 'NONE',  ( -422.6627218934914936, 399.9999999999998863, -141.4497041420118535 ) ) ;
#28462=DIRECTION ( 'NONE',  ( 1.000000000000000000, 1.850550996349095901E-16, 1.228197773518735191E-20 ) ) ;
#28464=ORIENTED_EDGE ( 'NONE', *, *, #43359, .F. ) ;
#28506=CARTESIAN_POINT ( 'NONE',  ( -442.6627218934912662, 394.9999999999998295, 103.5502958579880612 ) ) ;
#28509=DIRECTION ( 'NONE',  ( -1.000000000000000000, -3.697785493223490648E-32, 0.000000000000000000 ) ) ;
#28519=EDGE_CURVE ( 'NONE', #8171, #32531, #39966, .T. ) ;
#28529=CARTESIAN_POINT ( 'NONE',  ( 429.8372781065085633, 400.0000000000000568, -128.9497041420118251 ) ) ;
#28534=MECHANICAL_DESIGN_GEOMETRIC_PRESENTATION_REPRESENTATION('',(#36365),#57712);
#28537=LINE ( 'NONE', #44719, #16075 ) ;
#28573=EDGE_CURVE ( 'NONE', #58185, #41538, #2681, .T. ) ;
#28581=AXIS2_PLACEMENT_3D ( 'NONE', #66162, #11264, #64746 ) ;
#28607=DIRECTION ( 'NONE',  ( 1.000000000000000000, 0.000000000000000000, 0.000000000000000000 ) ) ;
#28613=DIRECTION ( 'NONE',  ( -1.850371928290090422E-16, 1.000000000000000000, 1.110223024625156171E-16 ) ) ;
#28618=DIRECTION ( 'NONE',  ( -1.020422603260505347E-14, 1.000000000000000000, 5.551115123125782702E-17 ) ) ;
#28641=ORIENTED_EDGE ( 'NONE', *, *, #44714, .F. ) ;
#28672=ORIENTED_EDGE ( 'NONE', *, *, #57352, .F. ) ;
#28696=ORIENTED_EDGE ( 'NONE', *, *, #40501, .F. ) ;
#28698=CARTESIAN_POINT ( 'NONE',  ( 412.3372781065085633, 179.4906275429376024, 111.5502958579881749 ) ) ;
#28703=CARTESIAN_POINT ( 'NONE',  ( -442.6627218934913230, 399.9999999999997726, 108.5502958579881891 ) ) ;
#28713=FACE_OUTER_BOUND ( 'NONE', #53561, .T. ) ;
#28770=ORIENTED_EDGE ( 'NONE', *, *, #54297, .T. ) ;
#28791=CARTESIAN_POINT ( 'NONE',  ( -442.6627218934912662, 394.9999999999998295, 113.5502958579881465 ) ) ;
#28793=AXIS2_PLACEMENT_3D ( 'NONE', #50392, #45803, #34216 ) ;
#28794=( LENGTH_UNIT ( ) NAMED_UNIT ( * ) SI_UNIT ( .MILLI., .METRE. ) );
#28810=CARTESIAN_POINT ( 'NONE',  ( 412.3372781065085633, 219.4906275429376308, 111.5502958579881749 ) ) ;
#28846=CARTESIAN_POINT ( 'NONE',  ( -452.6627218934913799, 0.000000000000000000, -146.4497041420118251 ) ) ;
#28850=VECTOR ( 'NONE', #17315, 1000.000000000000000 ) ;
#28867=CARTESIAN_POINT ( 'NONE',  ( -442.6627218934913230, 1.665334536937734811E-13, 108.5502958579881749 ) ) ;
#28892=ORIENTED_EDGE ( 'NONE', *, *, #31125, .F. ) ;
#28946=CARTESIAN_POINT ( 'NONE',  ( -447.6627218934913799, 0.000000000000000000, -136.4497041420118251 ) ) ;
#28984=ADVANCED_FACE ( 'NONE', ( #55983 ), #23966, .T. ) ;
#28992=( BOUNDED_CURVE ( )  B_SPLINE_CURVE ( 3, ( #21137, #59090, #53460, #43950 ),
 .UNSPECIFIED., .F., .F. ) 
 B_SPLINE_CURVE_WITH_KNOTS ( ( 4, 4 ),
 ( 4.791312937756477625E-14, 1.570796326794909437 ),
 .UNSPECIFIED. ) 
 CURVE ( )  GEOMETRIC_REPRESENTATION_ITEM ( )  RATIONAL_B_SPLINE_CURVE ( ( 1.000000000000000000, 0.8047378541243732641, 0.8047378541243732641, 1.000000000000000000 ) ) 
 REPRESENTATION_ITEM ( '' )  );
#28999=VECTOR ( 'NONE', #28036, 1000.000000000000000 ) ;
#29011=CARTESIAN_POINT ( 'NONE',  ( 437.3372781065085633, 395.0000000000001137, -146.4497041420118535 ) ) ;
#29033=CARTESIAN_POINT ( 'NONE',  ( -452.6627218934914367, 399.9999999999998863, -116.4497041420118393 ) ) ;
#29041=VECTOR ( 'NONE', #21719, 1000.000000000000114 ) ;
#29051=EDGE_LOOP ( 'NONE', ( #2604, #31053, #1247, #24935 ) ) ;
#29069=CARTESIAN_POINT ( 'NONE',  ( 433.3728120124416137, 388.0000000000066507, -132.4852380479447902 ) ) ;
#29078=CARTESIAN_POINT ( 'NONE',  ( -422.6627218934912662, 394.9999999999998295, 113.5502958579882034 ) ) ;
#29086=PLANE ( 'NONE',  #39675 ) ;
#29102=CARTESIAN_POINT ( 'NONE',  ( -417.6627218934913799, 399.9999999999998295, -111.4497041420118251 ) ) ;
#29125=EDGE_CURVE ( 'NONE', #34523, #17392, #38314, .T. ) ;
#29134=LINE ( 'NONE', #28791, #13778 ) ;
#29143=CARTESIAN_POINT ( 'NONE',  ( 433.3728120124415568, 395.0000000000042633, 99.58582976391699049 ) ) ;
#29147=SURFACE_SIDE_STYLE ('',( #40047 ) ) ;
#29155=DIRECTION ( 'NONE',  ( 0.000000000000000000, 1.000000000000000000, 0.000000000000000000 ) ) ;
#29203=CARTESIAN_POINT ( 'NONE',  ( 417.3372781065086201, 0.000000000000000000, -141.4497041420118251 ) ) ;
#29245=ORIENTED_EDGE ( 'NONE', *, *, #68894, .F. ) ;
#29250=CARTESIAN_POINT ( 'NONE',  ( 442.3372781065089612, 370.0000000000064801, -141.4497041420121661 ) ) ;
#29269=VECTOR ( 'NONE', #59576, 1000.000000000000000 ) ;
#29320=ADVANCED_FACE ( 'NONE', ( #957 ), #37896, .T. ) ;
#29332=VERTEX_POINT ( 'NONE', #27326 ) ;
#29340=DIRECTION ( 'NONE',  ( 6.405132834375901070E-16, -1.000000000000000000, -6.405132834375902056E-16 ) ) ;
#29354=CARTESIAN_POINT ( 'NONE',  ( -442.6627218934913230, 399.9999999999997726, 103.5502958579881891 ) ) ;
#29366=MECHANICAL_DESIGN_GEOMETRIC_PRESENTATION_REPRESENTATION('',(#2405),#48365);
#29367=CARTESIAN_POINT ( 'NONE',  ( -452.6627218934913230, 399.9999999999997726, 83.55029585798818914 ) ) ;
#29371=EDGE_CURVE ( 'NONE', #10959, #13791, #37860, .T. ) ;
#29429=ORIENTED_EDGE ( 'NONE', *, *, #51568, .T. ) ;
#29431=FACE_OUTER_BOUND ( 'NONE', #62979, .T. ) ;
#29476=SURFACE_SIDE_STYLE ('',( #8023 ) ) ;
#29502=LINE ( 'NONE', #18259, #61425 ) ;
#29508=CIRCLE ( 'NONE', #38488, 5.000000000000004441 ) ;
#29509=CARTESIAN_POINT ( 'NONE',  ( -7.662721893488489755, 395.0000000000064801, 308.5502958579854180 ) ) ;
#29510=LINE ( 'NONE', #50974, #25635 ) ;
#29513=CARTESIAN_POINT ( 'NONE',  ( -452.6627218934861503, 365.0000000000064233, -146.4497041420121377 ) ) ;
#29524=FACE_OUTER_BOUND ( 'NONE', #10619, .T. ) ;
#29544=DIRECTION ( 'NONE',  ( -1.000000000000000000, 0.000000000000000000, 7.703719777548943412E-34 ) ) ;
#29583=CYLINDRICAL_SURFACE ( 'NONE', #31662, 5.000000000000004441 ) ;
#29594=CARTESIAN_POINT ( 'NONE',  ( -452.6627218934913230, 399.9999999999998295, -146.4497041420117398 ) ) ;
#29597=VECTOR ( 'NONE', #23569, 1000.000000000000000 ) ;
#29613=CARTESIAN_POINT ( 'NONE',  ( 417.3372781065085633, 400.0000000000000568, -146.4497041420118535 ) ) ;
#29645=EDGE_CURVE ( 'NONE', #46683, #16988, #29502, .T. ) ;
#29648=CARTESIAN_POINT ( 'NONE',  ( 447.3372781065085064, 400.0000000000009663, -146.4497041420118535 ) ) ;
#29653=LINE ( 'NONE', #2925, #53362 ) ;
#29679=DIRECTION ( 'NONE',  ( -1.000000000000000000, 0.000000000000000000, -1.337618101958020291E-16 ) ) ;
#29684=CARTESIAN_POINT ( 'NONE',  ( 417.3372781065086770, 0.000000000000000000, 108.5502958579881749 ) ) ;
#29697=CIRCLE ( 'NONE', #61184, 5.000000000000004441 ) ;
#29739=VERTEX_POINT ( 'NONE', #35831 ) ;
#29759=DIRECTION ( 'NONE',  ( -4.270088556250601699E-16, -0.000000000000000000, -1.000000000000000000 ) ) ;
#29778=DIRECTION ( 'NONE',  ( -1.000000000000000000, -1.001918046209079887E-14, 9.729495617646301779E-15 ) ) ;
#29821=ORIENTED_EDGE ( 'NONE', *, *, #19628, .F. ) ;
#29822=ORIENTED_EDGE ( 'NONE', *, *, #53901, .T. ) ;
#29833=VECTOR ( 'NONE', #55778, 1000.000000000000000 ) ;
#29839=DIRECTION ( 'NONE',  ( -1.001915251000354105E-14, 1.000000000000000000, -5.551115123125782702E-17 ) ) ;
#29870=LINE ( 'NONE', #2791, #50374 ) ;
#29873=DIRECTION ( 'NONE',  ( -1.387778780781446169E-16, 1.000000000000000000, 3.469446951953615421E-17 ) ) ;
#29883=PLANE ( 'NONE',  #19564 ) ;
#29891=VERTEX_POINT ( 'NONE', #36863 ) ;
#29905=CARTESIAN_POINT ( 'NONE',  ( 442.3372781065085633, 369.9999999999999432, -141.4497041420118251 ) ) ;
#29922=ORIENTED_EDGE ( 'NONE', *, *, #48649, .F. ) ;
#29973=CARTESIAN_POINT ( 'NONE',  ( -452.6627218934913230, 217.8591479523843475, 78.55029585798814651 ) ) ;
#29979=VERTEX_POINT ( 'NONE', #46719 ) ;
#29982=VECTOR ( 'NONE', #37962, 1000.000000000000000 ) ;
#29984=CARTESIAN_POINT ( 'NONE',  ( -444.4229916354184979, 394.6798985497181889, -128.9497041420121093 ) ) ;
#29990=ORIENTED_EDGE ( 'NONE', *, *, #55999, .F. ) ;
#29997=LINE ( 'NONE', #63390, #25431 ) ;
#30031=PLANE ( 'NONE',  #15430 ) ;
#30057=ORIENTED_EDGE ( 'NONE', *, *, #56724, .T. ) ;
#30070=CARTESIAN_POINT ( 'NONE',  ( -452.6627218934913230, 177.8591479523843475, 78.55029585798814651 ) ) ;
#30104=LINE ( 'NONE', #46261, #7884 ) ;
#30111=ADVANCED_FACE ( 'NONE', ( #62735 ), #31077, .F. ) ;
#30138=ADVANCED_FACE ( 'NONE', ( #30373 ), #30031, .T. ) ;
#30147=VECTOR ( 'NONE', #27510, 1000.000000000000000 ) ;
#30175=ORIENTED_EDGE ( 'NONE', *, *, #8526, .F. ) ;
#30199=CARTESIAN_POINT ( 'NONE',  ( -444.4229916354184411, 400.0000000000065370, -128.9497041420121093 ) ) ;
#30220=EDGE_LOOP ( 'NONE', ( #6930, #64984, #42364, #58263 ) ) ;
#30228=FACE_OUTER_BOUND ( 'NONE', #5579, .T. ) ;
#30262=ORIENTED_EDGE ( 'NONE', *, *, #22943, .T. ) ;
#30270=LINE ( 'NONE', #37947, #36188 ) ;
#30281=CARTESIAN_POINT ( 'NONE',  ( -442.6627218934918915, 394.9999999999998295, -136.4497041420123367 ) ) ;
#30287=ORIENTED_EDGE ( 'NONE', *, *, #26512, .T. ) ;
#30288=ORIENTED_EDGE ( 'NONE', *, *, #16250, .T. ) ;
#30293=LINE ( 'NONE', #55987, #62227 ) ;
#30316=ORIENTED_EDGE ( 'NONE', *, *, #35755, .T. ) ;
#30321=ORIENTED_EDGE ( 'NONE', *, *, #51865, .T. ) ;
#30347=CARTESIAN_POINT ( 'NONE',  ( -447.6627218934914367, 399.9999999999998863, -116.4497041420118393 ) ) ;
#30358=DIRECTION ( 'NONE',  ( 1.000000000000000000, 1.387778780781445676E-16, 0.000000000000000000 ) ) ;
#30373=FACE_OUTER_BOUND ( 'NONE', #49893, .T. ) ;
#30383=DIRECTION ( 'NONE',  ( 1.000000000000000000, 0.000000000000000000, 0.000000000000000000 ) ) ;
#30415=DIRECTION ( 'NONE',  ( 9.729521452151193035E-15, -5.551115123116034723E-17, 1.000000000000000000 ) ) ;
#30439=EDGE_CURVE ( 'NONE', #65355, #9149, #25023, .T. ) ;
#30465=VECTOR ( 'NONE', #39016, 1000.000000000000000 ) ;
#30466=AXIS2_PLACEMENT_3D ( 'NONE', #22439, #33706, #60063 ) ;
#30469=VECTOR ( 'NONE', #16568, 1000.000000000000000 ) ;
#30472=LINE ( 'NONE', #34381, #18845 ) ;
#30488=DIRECTION ( 'NONE',  ( 1.000000000000000000, 1.024558601614476894E-14, -9.899298618516476860E-15 ) ) ;
#30515=( GEOMETRIC_REPRESENTATION_CONTEXT ( 3 ) GLOBAL_UNCERTAINTY_ASSIGNED_CONTEXT ( ( #19821 ) ) GLOBAL_UNIT_ASSIGNED_CONTEXT ( ( #69363, #31393, #31729 ) ) REPRESENTATION_CONTEXT ( 'NONE', 'WORKASPACE' ) );
#30525=DIRECTION ( 'NONE',  ( -1.000000000000000000, 2.279101714840934323E-64, -7.703719777548945123E-34 ) ) ;
#30532=EDGE_LOOP ( 'NONE', ( #51321, #31893, #65972, #26174 ) ) ;
#30584=ADVANCED_FACE ( 'NONE', ( #23209 ), #60480, .T. ) ;
#30593=LINE ( 'NONE', #20721, #7525 ) ;
#30623=( NAMED_UNIT ( * ) SI_UNIT ( $, .STERADIAN. ) SOLID_ANGLE_UNIT ( ) );
#30667=EDGE_CURVE ( 'NONE', #55132, #23082, #66475, .T. ) ;
#30678=LINE ( 'NONE', #4969, #61933 ) ;
#30683=CARTESIAN_POINT ( 'NONE',  ( -440.1146514826277212, 400.0000000000065370, -133.9016337311479958 ) ) ;
#30709=CARTESIAN_POINT ( 'NONE',  ( 444.4083459183738682, 365.0000000000043769, 110.6213636698493872 ) ) ;
#30739=CARTESIAN_POINT ( 'NONE',  ( -417.6627218934917778, 397.0710678118718988, -111.4497041420121519 ) ) ;
#30790=EDGE_CURVE ( 'NONE', #11742, #135, #29510, .T. ) ;
#30791=LINE ( 'NONE', #3702, #32606 ) ;
#30803=FACE_OUTER_BOUND ( 'NONE', #4836, .T. ) ;
#30804=DIRECTION ( 'NONE',  ( 1.000000000000000000, 1.132072239499580971E-16, -1.697513318603925187E-16 ) ) ;
#30835=ORIENTED_EDGE ( 'NONE', *, *, #35889, .F. ) ;
#30870=DIRECTION ( 'NONE',  ( 1.387778780781445429E-16, -1.000000000000000000, -3.081487911019577365E-33 ) ) ;
#30871=DIRECTION ( 'NONE',  ( -1.020422603260505347E-14, 1.000000000000000000, 5.551115123125782702E-17 ) ) ;
#30880=ORIENTED_EDGE ( 'NONE', *, *, #31094, .T. ) ;
#30906=EDGE_CURVE ( 'NONE', #9188, #57503, #11856, .T. ) ;
#30912=AXIS2_PLACEMENT_3D ( 'NONE', #36055, #57509, #9318 ) ;
#30927=DIRECTION ( 'NONE',  ( 1.020422603260505347E-14, -1.000000000000000000, -5.551115123125782702E-17 ) ) ;
#30939=DIRECTION ( 'NONE',  ( -1.000000000000000000, -6.405132834375901070E-16, -5.170250902511168442E-32 ) ) ;
#30941=ORIENTED_EDGE ( 'NONE', *, *, #44619, .F. ) ;
#30943=LINE ( 'NONE', #23931, #32090 ) ;
#30947=CARTESIAN_POINT ( 'NONE',  ( 447.3372781065085633, 365.0000000000001137, -146.4497041420118251 ) ) ;
#30953=VECTOR ( 'NONE', #15297, 1000.000000000000000 ) ;
#30957=AXIS2_PLACEMENT_3D ( 'NONE', #7980, #34021, #50543 ) ;
#30963=VECTOR ( 'NONE', #38535, 1000.000000000000000 ) ;
#30966=ADVANCED_FACE ( 'NONE', ( #18190 ), #39642, .F. ) ;
#30980=ORIENTED_EDGE ( 'NONE', *, *, #24880, .F. ) ;
#30998=VERTEX_POINT ( 'NONE', #51244 ) ;
#31046=VERTEX_POINT ( 'NONE', #67421 ) ;
#31051=ORIENTED_EDGE ( 'NONE', *, *, #56774, .T. ) ;
#31053=ORIENTED_EDGE ( 'NONE', *, *, #10466, .F. ) ;
#31077=CYLINDRICAL_SURFACE ( 'NONE', #14328, 5.000000000000004441 ) ;
#31094=EDGE_CURVE ( 'NONE', #15354, #48257, #30472, .T. ) ;
#31097=ORIENTED_EDGE ( 'NONE', *, *, #68485, .T. ) ;
#31125=EDGE_CURVE ( 'NONE', #41110, #11896, #52269, .T. ) ;
#31154=PRESENTATION_STYLE_ASSIGNMENT (( #35736 ) ) ;
#31158=ADVANCED_FACE ( 'NONE', ( #32536 ), #49396, .F. ) ;
#31161=AXIS2_PLACEMENT_3D ( 'NONE', #63544, #21311, #63885 ) ;
#31164=AXIS2_PLACEMENT_3D ( 'NONE', #22656, #65580, #17372 ) ;
#31185=ORIENTED_EDGE ( 'NONE', *, *, #42540, .F. ) ;
#31200=CARTESIAN_POINT ( 'NONE',  ( 412.3372781065085633, 179.4906275429376024, 113.5502958579881749 ) ) ;
#31232=( LENGTH_UNIT ( ) NAMED_UNIT ( * ) SI_UNIT ( .MILLI., .METRE. ) );
#31237=DIRECTION ( 'NONE',  ( -4.270088556250601699E-16, -0.000000000000000000, -1.000000000000000000 ) ) ;
#31251=( BOUNDED_CURVE ( )  B_SPLINE_CURVE ( 3, ( #15754, #57640, #10470, #47750 ),
 .UNSPECIFIED., .F., .F. ) 
 B_SPLINE_CURVE_WITH_KNOTS ( ( 4, 4 ),
 ( 1.570796326794897002, 3.141592653589793560 ),
 .UNSPECIFIED. ) 
 CURVE ( )  GEOMETRIC_REPRESENTATION_ITEM ( )  RATIONAL_B_SPLINE_CURVE ( ( 1.000000000000000000, 0.8047378541243649375, 0.8047378541243649375, 1.000000000000000000 ) ) 
 REPRESENTATION_ITEM ( '' )  );
#31266=CIRCLE ( 'NONE', #12174, 5.000000000000004441 ) ;
#31286=LINE ( 'NONE', #52715, #21547 ) ;
#31288=LINE ( 'NONE', #31971, #65927 ) ;
#31311=CARTESIAN_POINT ( 'NONE',  ( -417.6627218934913230, 219.4906275429376308, 113.5502958579881749 ) ) ;
#31324=DIRECTION ( 'NONE',  ( -1.850371928290090422E-16, 1.000000000000000000, 1.110223024625156171E-16 ) ) ;
#31327=ORIENTED_EDGE ( 'NONE', *, *, #52357, .T. ) ;
#31355=ORIENTED_EDGE ( 'NONE', *, *, #8078, .T. ) ;
#31369=CARTESIAN_POINT ( 'NONE',  ( -450.6627218934913230, 217.8591479523843475, -111.4497041420117966 ) ) ;
#31389=CARTESIAN_POINT ( 'NONE',  ( -442.9415673952016732, 394.9999999999997726, 92.47907109491421807 ) ) ;
#31393=( NAMED_UNIT ( * ) PLANE_ANGLE_UNIT ( ) SI_UNIT ( $, .RADIAN. ) );
#31403=EDGE_CURVE ( 'NONE', #22804, #49146, #19137, .T. ) ;
#31417=DIRECTION ( 'NONE',  ( -1.000000000000000000, 0.000000000000000000, 0.000000000000000000 ) ) ;
#31453=ADVANCED_FACE ( 'NONE', ( #5966 ), #48515, .T. ) ;
#31457=ORIENTED_EDGE ( 'NONE', *, *, #26351, .F. ) ;
#31471=LINE ( 'NONE', #492, #30953 ) ;
#31479=CARTESIAN_POINT ( 'NONE',  ( 437.3372781065085633, 400.0000000000000568, -141.4497041420118251 ) ) ;
#31506=DIRECTION ( 'NONE',  ( -0.7071067811865405783, -7.105427357601001070E-15, 0.7071067811865545671 ) ) ;
#31524=VECTOR ( 'NONE', #7883, 1000.000000000000000 ) ;
#31557=FACE_OUTER_BOUND ( 'NONE', #65439, .T. ) ;
#31562=VECTOR ( 'NONE', #37924, 1000.000000000000000 ) ;
#31612=CARTESIAN_POINT ( 'NONE',  ( -452.6627218934860934, 395.0000000000064801, -133.9497041420121377 ) ) ;
#31616=EDGE_LOOP ( 'NONE', ( #36249, #20541, #8557, #28696 ) ) ;
#31623=DIRECTION ( 'NONE',  ( 4.314083075427411048E-32, 1.000000000000000000, 6.123233995736763571E-17 ) ) ;
#31629=ORIENTED_EDGE ( 'NONE', *, *, #69550, .F. ) ;
#31641=CARTESIAN_POINT ( 'NONE',  ( 429.8372781065087906, 388.0000000000109708, 101.0502958579843806 ) ) ;
#31645=( NAMED_UNIT ( * ) PLANE_ANGLE_UNIT ( ) SI_UNIT ( $, .RADIAN. ) );
#31662=AXIS2_PLACEMENT_3D ( 'NONE', #12723, #61937, #23631 ) ;
#31665=AXIS2_PLACEMENT_3D ( 'NONE', #52037, #57669, #41832 ) ;
#31729=( NAMED_UNIT ( * ) SI_UNIT ( $, .STERADIAN. ) SOLID_ANGLE_UNIT ( ) );
#31741=LINE ( 'NONE', #1736, #37399 ) ;
#31753=CARTESIAN_POINT ( 'NONE',  ( 412.3372781065086201, 400.0000000000000568, -146.4497041420118251 ) ) ;
#31754=FACE_OUTER_BOUND ( 'NONE', #2145, .T. ) ;
#31761=ORIENTED_EDGE ( 'NONE', *, *, #19628, .T. ) ;
#31786=CARTESIAN_POINT ( 'NONE',  ( -439.4229916354183842, 400.0000000000065370, -123.9497041420119530 ) ) ;
#31800=AXIS2_PLACEMENT_3D ( 'NONE', #49091, #929, #18154 ) ;
#31804=CARTESIAN_POINT ( 'NONE',  ( -317.6627218934913230, 394.9999999999997158, -11.44970414201176823 ) ) ;
#31806=CARTESIAN_POINT ( 'NONE',  ( -417.6627218934913230, 179.4906275429376308, -144.4497041420118819 ) ) ;
#31830=CARTESIAN_POINT ( 'NONE',  ( 447.3372781065086201, 400.0000000000044338, 113.5502958579838122 ) ) ;
#31839=ADVANCED_FACE ( 'NONE', ( #30228 ), #24610, .T. ) ;
#31867=AXIS2_PLACEMENT_3D ( 'NONE', #64529, #27234, #508 ) ;
#31889=AXIS2_PLACEMENT_3D ( 'NONE', #58065, #25380, #62303 ) ;
#31893=ORIENTED_EDGE ( 'NONE', *, *, #15818, .F. ) ;
#31894=ORIENTED_EDGE ( 'NONE', *, *, #36201, .F. ) ;
#31905=VECTOR ( 'NONE', #27739, 1000.000000000000114 ) ;
#31971=CARTESIAN_POINT ( 'NONE',  ( 112.3013380801406100, 400.0000000000077307, 91.05029585798746439 ) ) ;
#31992=ADVANCED_FACE ( 'NONE', ( #49486 ), #27695, .T. ) ;
#32023=CARTESIAN_POINT ( 'NONE',  ( -430.1627218934916641, 395.0000000000064801, -123.9497041420119530 ) ) ;
#32050=AXIS2_PLACEMENT_3D ( 'NONE', #17341, #18050, #28607 ) ;
#32075=ORIENTED_EDGE ( 'NONE', *, *, #54050, .F. ) ;
#32079=CARTESIAN_POINT ( 'NONE',  ( -447.6627218934918346, 367.0710678118609280, 108.5502958579925519 ) ) ;
#32090=VECTOR ( 'NONE', #45381, 1000.000000000000114 ) ;
#32091=CARTESIAN_POINT ( 'NONE',  ( -452.6627218934913230, 177.8591479523843475, 78.55029585798814651 ) ) ;
#32116=DIRECTION ( 'NONE',  ( 1.000000000000000000, 0.000000000000000000, 0.000000000000000000 ) ) ;
#32117=DIRECTION ( 'NONE',  ( 1.000000000000000000, 0.000000000000000000, 0.000000000000000000 ) ) ;
#32147=VERTEX_POINT ( 'NONE', #6599 ) ;
#32181=EDGE_CURVE ( 'NONE', #15124, #41255, #60506, .T. ) ;
#32233=LINE ( 'NONE', #48373, #22160 ) ;
#32262=VECTOR ( 'NONE', #21246, 1000.000000000000000 ) ;
#32293=CARTESIAN_POINT ( 'NONE',  ( -439.4229916354182706, 394.9999999999998295, -123.9497041420119530 ) ) ;
#32313=FACE_OUTER_BOUND ( 'NONE', #37588, .T. ) ;
#32321=CARTESIAN_POINT ( 'NONE',  ( -422.6627218934913230, 1.665334536937734811E-13, 113.5502958579881749 ) ) ;
#32333=AXIS2_PLACEMENT_3D ( 'NONE', #26246, #63528, #63875 ) ;
#32335=PLANE ( 'NONE',  #3362 ) ;
#32339=CIRCLE ( 'NONE', #34622, 5.000000000000004441 ) ;
#32346=CARTESIAN_POINT ( 'NONE',  ( 412.3372781065085633, 397.0710678118654755, -111.4497041420117824 ) ) ;
#32350=VECTOR ( 'NONE', #28509, 1000.000000000000000 ) ;
#32374=DIRECTION ( 'NONE',  ( 0.000000000000000000, -1.000000000000000000, -1.110223024625156171E-16 ) ) ;
#32377=PLANE ( 'NONE',  #40170 ) ;
#32394=VECTOR ( 'NONE', #56782, 1000.000000000000000 ) ;
#32403=DIRECTION ( 'NONE',  ( 0.000000000000000000, -1.000000000000000000, 1.479221584281239571E-31 ) ) ;
#32451=DIRECTION ( 'NONE',  ( 1.000000000000000000, -9.109522253334613014E-16, 0.000000000000000000 ) ) ;
#32459=CARTESIAN_POINT ( 'NONE',  ( 417.3372781065085633, 400.0000000000000568, -146.4497041420118251 ) ) ;
#32460=ORIENTED_EDGE ( 'NONE', *, *, #49625, .T. ) ;
#32464=VERTEX_POINT ( 'NONE', #540 ) ;
#32506=AXIS2_PLACEMENT_3D ( 'NONE', #18920, #37158, #5153 ) ;
#32509=CARTESIAN_POINT ( 'NONE',  ( 445.3372781065085633, 217.8591479523844612, -111.4497041420119388 ) ) ;
#32526=DIRECTION ( 'NONE',  ( 0.7071067811865476838, -5.551115123125782086E-17, 0.7071067811865473507 ) ) ;
#32527=CARTESIAN_POINT ( 'NONE',  ( -443.6249203811465804, 394.9114286947786354, -131.6832696988547298 ) ) ;
#32531=VERTEX_POINT ( 'NONE', #50814 ) ;
#32536=FACE_OUTER_BOUND ( 'NONE', #11292, .T. ) ;
#32551=CARTESIAN_POINT ( 'NONE',  ( 424.8372781065088475, 395.0000000000001137, -123.9497041420121235 ) ) ;
#32562=ORIENTED_EDGE ( 'NONE', *, *, #44830, .F. ) ;
#32595=DIRECTION ( 'NONE',  ( -1.850169831522831466E-16, 1.000000000000000000, 1.110223024625156294E-16 ) ) ;
#32606=VECTOR ( 'NONE', #14267, 1000.000000000000000 ) ;
#32677=DIRECTION ( 'NONE',  ( -1.850371928290090422E-16, 1.000000000000000000, 1.110223024625156171E-16 ) ) ;
#32687=DIRECTION ( 'NONE',  ( -1.000000000000000000, 0.000000000000000000, -0.000000000000000000 ) ) ;
#32726=COLOUR_RGB ( '',0.7921568627450980005, 0.8196078431372548767, 0.9333333333333333481 ) ;
#32735=CARTESIAN_POINT ( 'NONE',  ( -447.6627218934913230, 392.9289321881344108, 108.5502958579880328 ) ) ;
#32748=VERTEX_POINT ( 'NONE', #15943 ) ;
#32761=AXIS2_PLACEMENT_3D ( 'NONE', #37285, #16182, #59431 ) ;
#32807=ORIENTED_EDGE ( 'NONE', *, *, #20089, .F. ) ;
#32833=ORIENTED_EDGE ( 'NONE', *, *, #6822, .F. ) ;
#32851=EDGE_CURVE ( 'NONE', #35076, #26400, #27180, .T. ) ;
#32901=PLANE ( 'NONE',  #55199 ) ;
#32913=VECTOR ( 'NONE', #65563, 1000.000000000000000 ) ;
#32953=LINE ( 'NONE', #54392, #61187 ) ;
#32975=PLANE ( 'NONE',  #66103 ) ;
#32979=CARTESIAN_POINT ( 'NONE',  ( -452.6627218934913230, 0.000000000000000000, -6.938893903907228378E-15 ) ) ;
#32996=ORIENTED_EDGE ( 'NONE', *, *, #32181, .T. ) ;
#33013=ORIENTED_EDGE ( 'NONE', *, *, #37162, .T. ) ;
#33021=CARTESIAN_POINT ( 'NONE',  ( -447.6627218934913230, 399.9999999999997726, 103.5502958579881891 ) ) ;
#33024=ADVANCED_FACE ( 'NONE', ( #329 ), #21782, .F. ) ;
#33039=CARTESIAN_POINT ( 'NONE',  ( -317.6627218934913230, 394.9999999999997158, -11.44970414201176823 ) ) ;
#33056=EDGE_CURVE ( 'NONE', #62663, #28396, #57922, .T. ) ;
#33059=EDGE_LOOP ( 'NONE', ( #63319, #46185, #54568, #7983 ) ) ;
#33096=FACE_OUTER_BOUND ( 'NONE', #44226, .T. ) ;
#33106=CARTESIAN_POINT ( 'NONE',  ( -447.6627218934913230, 394.9999999999998295, 108.5502958579881181 ) ) ;
#33123=CARTESIAN_POINT ( 'NONE',  ( -444.1126562889743923, 394.7876926391177790, 94.27943548784956818 ) ) ;
#33138=CARTESIAN_POINT ( 'NONE',  ( 442.3372781065083359, 370.0000000000043201, 108.5502958579838833 ) ) ;
#33152=VECTOR ( 'NONE', #67704, 1000.000000000000000 ) ;
#33153=ORIENTED_EDGE ( 'NONE', *, *, #56875, .T. ) ;
#33160=LINE ( 'NONE', #18022, #28850 ) ;
#33167=ORIENTED_EDGE ( 'NONE', *, *, #9454, .F. ) ;
#33170=DIRECTION ( 'NONE',  ( -1.020422603260505347E-14, 1.000000000000000000, 5.551115123125782702E-17 ) ) ;
#33228=APPLICATION_CONTEXT ( 'automotive_design' ) ;
#33255=ORIENTED_EDGE ( 'NONE', *, *, #68983, .F. ) ;
#33321=DIRECTION ( 'NONE',  ( -1.000000000000000000, 0.000000000000000000, 0.000000000000000000 ) ) ;
#33341=CARTESIAN_POINT ( 'NONE',  ( -419.7337897053568554, 394.9999999999998863, -113.5207719538772579 ) ) ;
#33355=VERTEX_POINT ( 'NONE', #7228 ) ;
#33385=DIRECTION ( 'NONE',  ( 1.000000000000000000, 0.000000000000000000, -2.921639538487254261E-16 ) ) ;
#33425=AXIS2_PLACEMENT_3D ( 'NONE', #64151, #27552, #11369 ) ;
#33432=DIRECTION ( 'NONE',  ( -1.850371928290090422E-16, 1.000000000000000000, 1.110223024625156171E-16 ) ) ;
#33444=FACE_OUTER_BOUND ( 'NONE', #45481, .T. ) ;
#33447=DIRECTION ( 'NONE',  ( -1.387778780781446169E-16, 1.000000000000000000, 3.469446951953615421E-17 ) ) ;
#33457=CARTESIAN_POINT ( 'NONE',  ( -417.6627218934913230, 399.9999999999998295, 78.55029585798814651 ) ) ;
#33469=FILL_AREA_STYLE ('',( #43986 ) ) ;
#33480=DIRECTION ( 'NONE',  ( 1.387778780781446169E-16, -1.000000000000000000, -3.469446951953615421E-17 ) ) ;
#33481=EDGE_LOOP ( 'NONE', ( #50958, #66320, #42674, #36788 ) ) ;
#33546=ORIENTED_EDGE ( 'NONE', *, *, #47955, .F. ) ;
#33547=ORIENTED_EDGE ( 'NONE', *, *, #43310, .F. ) ;
#33559=CARTESIAN_POINT ( 'NONE',  ( 50.98853755884148597, 388.0000000000071054, 96.05029585798814651 ) ) ;
#33570=( GEOMETRIC_REPRESENTATION_CONTEXT ( 3 ) GLOBAL_UNCERTAINTY_ASSIGNED_CONTEXT ( ( #60643 ) ) GLOBAL_UNIT_ASSIGNED_CONTEXT ( ( #59043, #43203, #21759 ) ) REPRESENTATION_CONTEXT ( 'NONE', 'WORKASPACE' ) );
#33574=ORIENTED_EDGE ( 'NONE', *, *, #56822, .T. ) ;
#33592=EDGE_CURVE ( 'NONE', #45368, #3161, #10326, .T. ) ;
#33625=CARTESIAN_POINT ( 'NONE',  ( 107.3013380801407521, 388.0000000000076739, 96.05029585798752123 ) ) ;
#33646=CARTESIAN_POINT ( 'NONE',  ( 433.3728120124415568, 394.9999999999999432, 99.58582976392126795 ) ) ;
#33664=LINE ( 'NONE', #61759, #24804 ) ;
#33674=CARTESIAN_POINT ( 'NONE',  ( -439.4229916354184411, 388.0000000000020464, 96.05029585799300662 ) ) ;
#33706=DIRECTION ( 'NONE',  ( 1.850169831522831466E-16, -1.000000000000000000, 5.551115123125781470E-17 ) ) ;
#33711=VECTOR ( 'NONE', #7822, 1000.000000000000000 ) ;
#33712=DIRECTION ( 'NONE',  ( 1.387778780781445922E-16, -1.000000000000000000, -1.232595164407830946E-32 ) ) ;
#33740=VECTOR ( 'NONE', #46529, 1000.000000000000000 ) ;
#33749=DIRECTION ( 'NONE',  ( 0.7071067811865475727, 2.220446049250312341E-16, -0.7071067811865474617 ) ) ;
#33752=DIRECTION ( 'NONE',  ( -1.850169831522831466E-16, 1.000000000000000000, 1.110223024625156294E-16 ) ) ;
#33772=CARTESIAN_POINT ( 'NONE',  ( -422.6627218934913230, 399.9999999999997726, 113.5502958579881891 ) ) ;
#33773=LINE ( 'NONE', #11957, #13727 ) ;
#33774=CARTESIAN_POINT ( 'NONE',  ( 412.3372781065085633, 219.4906275429376308, -146.4497041420117682 ) ) ;
#33778=VERTEX_POINT ( 'NONE', #46848 ) ;
#33782=ORIENTED_EDGE ( 'NONE', *, *, #68309, .T. ) ;
#33826=EDGE_LOOP ( 'NONE', ( #60897, #18023, #62818, #1868, #2311, #21539, #57896 ) ) ;
#33827=EDGE_LOOP ( 'NONE', ( #59627, #22118, #20286, #23676 ) ) ;
#33835=EDGE_CURVE ( 'NONE', #68286, #21636, #65827, .T. ) ;
#33869=LINE ( 'NONE', #23663, #61809 ) ;
#33874=ORIENTED_EDGE ( 'NONE', *, *, #16969, .T. ) ;
#33876=AXIS2_PLACEMENT_3D ( 'NONE', #11275, #65104, #21831 ) ;
#33887=STYLED_ITEM ( 'NONE', ( #10610 ), #16524 ) ;
#33915=DIRECTION ( 'NONE',  ( 0.7071067811865474617, 0.000000000000000000, -0.7071067811865476838 ) ) ;
#33944=EDGE_CURVE ( 'NONE', #68395, #27359, #67209, .T. ) ;
#33947=DIRECTION ( 'NONE',  ( -0.000000000000000000, 0.000000000000000000, -1.000000000000000000 ) ) ;
#33961=ORIENTED_EDGE ( 'NONE', *, *, #34428, .F. ) ;
#33965=LINE ( 'NONE', #33625, #45517 ) ;
#33986=CIRCLE ( 'NONE', #3649, 5.000000000000004441 ) ;
#33989=DIRECTION ( 'NONE',  ( -3.081487911019579554E-32, -1.000000000000000000, -3.469446951953612956E-17 ) ) ;
#33995=EDGE_CURVE ( 'NONE', #10801, #41137, #11273, .T. ) ;
#33996=ORIENTED_EDGE ( 'NONE', *, *, #14295, .T. ) ;
#34012=PLANE ( 'NONE',  #36318 ) ;
#34021=DIRECTION ( 'NONE',  ( -4.314083075427411048E-32, -1.000000000000000000, -6.123233995736762338E-17 ) ) ;
#34022=EDGE_CURVE ( 'NONE', #54476, #41255, #5994, .T. ) ;
#34023=CARTESIAN_POINT ( 'NONE',  ( 299.8372781065085064, 399.9999999999998863, -33.94970414201181796 ) ) ;
#34035=ORIENTED_EDGE ( 'NONE', *, *, #15008, .T. ) ;
#34038=CARTESIAN_POINT ( 'NONE',  ( 447.3372781065086770, 400.0000000000066507, -146.4497041420121093 ) ) ;
#34097=CARTESIAN_POINT ( 'NONE',  ( -439.4229916354184979, 400.0000000000065370, -133.9497041420121377 ) ) ;
#34100=DIRECTION ( 'NONE',  ( 1.000000000000000000, 1.387778780781448634E-16, -1.387778780781445676E-15 ) ) ;
#34114=EDGE_CURVE ( 'NONE', #35973, #13434, #38416, .T. ) ;
#34116=CARTESIAN_POINT ( 'NONE',  ( -452.6627218934859798, 400.0000000000064801, -146.4497041420121377 ) ) ;
#34188=CARTESIAN_POINT ( 'NONE',  ( -447.6627218934913799, 0.000000000000000000, -116.4497041420118393 ) ) ;
#34216=DIRECTION ( 'NONE',  ( 1.604841615724182364E-15, 1.000000000000000000, 0.000000000000000000 ) ) ;
#34219=VERTEX_POINT ( 'NONE', #53750 ) ;
#34255=DIRECTION ( 'NONE',  ( 0.000000000000000000, 1.232595164407830672E-32, 1.000000000000000000 ) ) ;
#34289=FACE_OUTER_BOUND ( 'NONE', #34295, .T. ) ;
#34295=EDGE_LOOP ( 'NONE', ( #63046, #228, #68307, #37874 ) ) ;
#34305=EDGE_LOOP ( 'NONE', ( #15002, #35007, #32833, #56878 ) ) ;
#34366=CARTESIAN_POINT ( 'NONE',  ( 447.3372781065085633, 400.0000000000000568, -116.4497041420118393 ) ) ;
#34380=CARTESIAN_POINT ( 'NONE',  ( 447.3372781065086201, 217.8591479523844612, 78.55029585798806124 ) ) ;
#34381=CARTESIAN_POINT ( 'NONE',  ( -447.6627218934889925, 395.0000000000064801, -141.4497041420092387 ) ) ;
#34428=EDGE_CURVE ( 'NONE', #135, #2857, #23856, .T. ) ;
#34434=EDGE_CURVE ( 'NONE', #36808, #26715, #62849, .T. ) ;
#34445=FILL_AREA_STYLE ('',( #51644 ) ) ;
#34451=CARTESIAN_POINT ( 'NONE',  ( 50.98853755884148597, 395.0000000000004547, 101.0502958579881465 ) ) ;
#34486=LINE ( 'NONE', #64689, #11658 ) ;
#34512=ORIENTED_EDGE ( 'NONE', *, *, #52639, .T. ) ;
#34514=CARTESIAN_POINT ( 'NONE',  ( 417.3372781065086770, 0.000000000000000000, 113.5502958579881749 ) ) ;
#34519=DIRECTION ( 'NONE',  ( -1.232595164407830946E-32, -1.000000000000000000, 1.479221584281239571E-31 ) ) ;
#34523=VERTEX_POINT ( 'NONE', #63557 ) ;
#34561=DIRECTION ( 'NONE',  ( -2.612346171088249236E-15, -1.000000000000000000, 7.216449660063517513E-16 ) ) ;
#34573=DIRECTION ( 'NONE',  ( 0.000000000000000000, -1.000000000000000000, 0.000000000000000000 ) ) ;
#34601=DIRECTION ( 'NONE',  ( -1.000000000000000000, 0.000000000000000000, 0.000000000000000000 ) ) ;
#34610=EDGE_LOOP ( 'NONE', ( #4921, #48815, #34865, #46157 ) ) ;
#34622=AXIS2_PLACEMENT_3D ( 'NONE', #49024, #6124, #55722 ) ;
#34678=MECHANICAL_DESIGN_GEOMETRIC_PRESENTATION_REPRESENTATION('',(#5476),#4339);
#34682=DIRECTION ( 'NONE',  ( -1.850371928290090422E-16, 1.000000000000000000, 1.110223024625156294E-16 ) ) ;
#34688=ORIENTED_EDGE ( 'NONE', *, *, #59678, .F. ) ;
#34711=VERTEX_POINT ( 'NONE', #57418 ) ;
#34713=CARTESIAN_POINT ( 'NONE',  ( 442.3372781065085633, 400.0000000000000568, -136.4497041420118251 ) ) ;
#34767=VECTOR ( 'NONE', #62404, 1000.000000000000000 ) ;
#34784=PRESENTATION_STYLE_ASSIGNMENT (( #66805 ) ) ;
#34789=DIRECTION ( 'NONE',  ( -0.7071067811865476838, -1.110223024625156294E-16, -0.7071067811865474617 ) ) ;
#34790=LINE ( 'NONE', #34097, #61096 ) ;
#34795=VERTEX_POINT ( 'NONE', #42615 ) ;
#34804=ADVANCED_FACE ( 'NONE', ( #5661 ), #48216, .T. ) ;
#34814=DIRECTION ( 'NONE',  ( -1.000000000000000000, 0.000000000000000000, 0.000000000000000000 ) ) ;
#34831=CARTESIAN_POINT ( 'NONE',  ( -452.6627218934859798, 400.0000000000064801, -146.4497041420121377 ) ) ;
#34865=ORIENTED_EDGE ( 'NONE', *, *, #24252, .F. ) ;
#34878=CARTESIAN_POINT ( 'NONE',  ( 447.3372781065085633, 365.0000000000001137, -146.4497041420116261 ) ) ;
#34907=VERTEX_POINT ( 'NONE', #55602 ) ;
#34926=ORIENTED_EDGE ( 'NONE', *, *, #64905, .T. ) ;
#34958=DIRECTION ( 'NONE',  ( -1.850169831522831466E-16, 1.000000000000000000, 1.110223024625156294E-16 ) ) ;
#34960=ADVANCED_FACE ( 'NONE', ( #60535 ), #8112, .T. ) ;
#34963=CARTESIAN_POINT ( 'NONE',  ( -439.4229916354182706, 394.9999999999998295, 91.05029585798840230 ) ) ;
#35004=LINE ( 'NONE', #67371, #38275 ) ;
#35006=CARTESIAN_POINT ( 'NONE',  ( 50.98853755884157835, 388.0000000000065370, -128.9497041420121946 ) ) ;
#35007=ORIENTED_EDGE ( 'NONE', *, *, #40793, .F. ) ;
#35014=CARTESIAN_POINT ( 'NONE',  ( 442.3372781065086201, 0.000000000000000000, 103.5502958579881749 ) ) ;
#35036=VECTOR ( 'NONE', #9315, 1000.000000000000000 ) ;
#35076=VERTEX_POINT ( 'NONE', #19354 ) ;
#35088=EDGE_LOOP ( 'NONE', ( #3450, #57049, #43356, #29822 ) ) ;
#35100=CYLINDRICAL_SURFACE ( 'NONE', #69232, 5.000000000000004441 ) ;
#35106=CARTESIAN_POINT ( 'NONE',  ( -447.6627218934912662, 369.9999999999998863, 108.5502958579877060 ) ) ;
#35110=EDGE_LOOP ( 'NONE', ( #42576, #32075, #39320, #52970, #67290, #49406, #26233 ) ) ;
#35124=ORIENTED_EDGE ( 'NONE', *, *, #69550, .T. ) ;
#35157=ORIENTED_EDGE ( 'NONE', *, *, #28276, .F. ) ;
#35198=CARTESIAN_POINT ( 'NONE',  ( 417.3372781065086201, 399.9999999999998863, 108.5502958579881891 ) ) ;
#35208=CARTESIAN_POINT ( 'NONE',  ( 447.3372781065086201, 0.000000000000000000, -146.4497041420118251 ) ) ;
#35216=CIRCLE ( 'NONE', #54254, 5.000000000000004441 ) ;
#35217=CARTESIAN_POINT ( 'NONE',  ( -442.6627218934914367, 399.9999999999998863, -136.4497041420118251 ) ) ;
#35233=CIRCLE ( 'NONE', #31867, 5.000000000000087930 ) ;
#35260=CARTESIAN_POINT ( 'NONE',  ( -442.6627218934913799, 394.9999999999998295, -125.1412729879898791 ) ) ;
#35271=CARTESIAN_POINT ( 'NONE',  ( -452.6627218934861503, 370.0000000000064233, -146.4497041420121377 ) ) ;
#35301=CARTESIAN_POINT ( 'NONE',  ( 50.98853755884139360, 388.0000000000071054, 91.05029585798797598 ) ) ;
#35302=CARTESIAN_POINT ( 'NONE',  ( -452.6627218934913799, 0.000000000000000000, -111.4497041420118251 ) ) ;
#35306=DIRECTION ( 'NONE',  ( 0.000000000000000000, -1.000000000000000000, 0.000000000000000000 ) ) ;
#35325=ORIENTED_EDGE ( 'NONE', *, *, #6822, .T. ) ;
#35353=DIRECTION ( 'NONE',  ( -1.850169831522831466E-16, 1.000000000000000000, 1.110223024625156294E-16 ) ) ;
#35366=AXIS2_PLACEMENT_3D ( 'NONE', #32321, #31623, #57677 ) ;
#35396=DIRECTION ( 'NONE',  ( 1.000000000000000000, 0.000000000000000000, 0.000000000000000000 ) ) ;
#35407=ORIENTED_EDGE ( 'NONE', *, *, #21449, .F. ) ;
#35460=VECTOR ( 'NONE', #37850, 1000.000000000000000 ) ;
#35467=VECTOR ( 'NONE', #48830, 1000.000000000000000 ) ;
#35476=ORIENTED_EDGE ( 'NONE', *, *, #48256, .F. ) ;
#35496=EDGE_CURVE ( 'NONE', #65265, #12369, #62880, .T. ) ;
#35515=AXIS2_PLACEMENT_3D ( 'NONE', #25952, #62552, #14362 ) ;
#35553=PRESENTATION_STYLE_ASSIGNMENT (( #20395 ) ) ;
#35559=FACE_OUTER_BOUND ( 'NONE', #14734, .T. ) ;
#35573=VECTOR ( 'NONE', #27955, 1000.000000000000000 ) ;
#35574=ORIENTED_EDGE ( 'NONE', *, *, #61789, .F. ) ;
#35625=LINE ( 'NONE', #57078, #16418 ) ;
#35649=ORIENTED_EDGE ( 'NONE', *, *, #56243, .T. ) ;
#35651=EDGE_CURVE ( 'NONE', #28296, #68802, #30791, .T. ) ;
#35667=ADVANCED_FACE ( 'NONE', ( #46260 ), #2331, .F. ) ;
#35670=ADVANCED_FACE ( 'NONE', ( #24821 ), #40997, .T. ) ;
#35671=ORIENTED_EDGE ( 'NONE', *, *, #50583, .F. ) ;
#35676=DIRECTION ( 'NONE',  ( 1.387778780781445429E-16, -1.000000000000000000, -3.081487911019577365E-33 ) ) ;
#35683=CARTESIAN_POINT ( 'NONE',  ( 447.3372781065086201, 400.0000000000044338, 113.5502958579838122 ) ) ;
#35705=CARTESIAN_POINT ( 'NONE',  ( 424.8372781065087906, 400.0000000000109139, 91.05029585798442326 ) ) ;
#35722=VECTOR ( 'NONE', #18271, 1000.000000000000000 ) ;
#35736=SURFACE_STYLE_USAGE ( .BOTH. , #62807 ) ;
#35755=EDGE_CURVE ( 'NONE', #15022, #20970, #41683, .T. ) ;
#35778=CARTESIAN_POINT ( 'NONE',  ( -447.6627218934913230, 1.665334536937734811E-13, 83.55029585798817493 ) ) ;
#35783=ORIENTED_EDGE ( 'NONE', *, *, #63831, .T. ) ;
#35797=EDGE_LOOP ( 'NONE', ( #3582, #4963, #61848, #2983, #41604, #40384, #61094 ) ) ;
#35803=FACE_OUTER_BOUND ( 'NONE', #67490, .T. ) ;
#35807=CARTESIAN_POINT ( 'NONE',  ( -447.6627218934916073, 370.0000000000085265, 108.5502958579925377 ) ) ;
#35816=ORIENTED_EDGE ( 'NONE', *, *, #48500, .T. ) ;
#35819=CARTESIAN_POINT ( 'NONE',  ( 447.3372781065085633, 400.0000000000000568, -146.4497041420118251 ) ) ;
#35831=CARTESIAN_POINT ( 'NONE',  ( -452.6627218934913230, 217.8591479523843475, -111.4497041420117966 ) ) ;
#35867=DIRECTION ( 'NONE',  ( 7.703719777548945123E-34, 1.479221584281240009E-31, -1.000000000000000000 ) ) ;
#35889=EDGE_CURVE ( 'NONE', #68707, #38702, #43047, .T. ) ;
#35901=CARTESIAN_POINT ( 'NONE',  ( 412.3372781065082791, 400.0000000000040927, 78.55029585798418168 ) ) ;
#35917=ORIENTED_EDGE ( 'NONE', *, *, #46850, .T. ) ;
#35925=ORIENTED_EDGE ( 'NONE', *, *, #11540, .T. ) ;
#35926=ORIENTED_EDGE ( 'NONE', *, *, #788, .F. ) ;
#35962=DIRECTION ( 'NONE',  ( -1.387778780781445429E-16, 1.000000000000000000, 3.081487911019577365E-33 ) ) ;
#35973=VERTEX_POINT ( 'NONE', #22648 ) ;
#35979=LINE ( 'NONE', #46878, #4293 ) ;
#36008=EDGE_LOOP ( 'NONE', ( #25362, #60971, #48852, #10886 ) ) ;
#36012=CARTESIAN_POINT ( 'NONE',  ( -422.6627218934918915, 395.0000000000064801, -116.4497041420121377 ) ) ;
#36015=VERTEX_POINT ( 'NONE', #1541 ) ;
#36047=EDGE_LOOP ( 'NONE', ( #20922, #54655, #62725, #7846 ) ) ;
#36055=CARTESIAN_POINT ( 'NONE',  ( -417.6627218934913230, 219.4906275429376308, 111.5502958579881749 ) ) ;
#36058=ORIENTED_EDGE ( 'NONE', *, *, #65508, .T. ) ;
#36072=SURFACE_STYLE_FILL_AREA ( #25870 ) ;
#36104=VERTEX_POINT ( 'NONE', #41266 ) ;
#36108=ORIENTED_EDGE ( 'NONE', *, *, #26512, .F. ) ;
#36116=CARTESIAN_POINT ( 'NONE',  ( -439.4229916354183842, 400.0000000000021032, 101.0502958579930066 ) ) ;
#36127=CIRCLE ( 'NONE', #49606, 5.000000000000170530 ) ;
#36164=ORIENTED_EDGE ( 'NONE', *, *, #15864, .F. ) ;
#36188=VECTOR ( 'NONE', #43905, 1000.000000000000000 ) ;
#36201=EDGE_CURVE ( 'NONE', #23006, #59231, #24049, .T. ) ;
#36205=EDGE_CURVE ( 'NONE', #63860, #52163, #54111, .T. ) ;
#36215=PLANE ( 'NONE',  #68059 ) ;
#36223=DIRECTION ( 'NONE',  ( -1.000000000000000000, -3.697785493223490648E-32, 0.000000000000000000 ) ) ;
#36224=EDGE_CURVE ( 'NONE', #22804, #36796, #43744, .T. ) ;
#36249=ORIENTED_EDGE ( 'NONE', *, *, #65706, .T. ) ;
#36263=PRESENTATION_STYLE_ASSIGNMENT (( #26059 ) ) ;
#36278=CARTESIAN_POINT ( 'NONE',  ( 412.3372781065085633, 179.4906275429376024, 111.5502958579881749 ) ) ;
#36318=AXIS2_PLACEMENT_3D ( 'NONE', #67410, #45246, #51229 ) ;
#36324=CARTESIAN_POINT ( 'NONE',  ( -439.4229916354182706, 388.0000000000064801, -123.9497041420119530 ) ) ;
#36356=CARTESIAN_POINT ( 'NONE',  ( 447.3372781065085633, 400.0000000000000568, -111.4497041420118251 ) ) ;
#36365=STYLED_ITEM ( 'NONE', ( #36263 ), #41747 ) ;
#36372=STYLED_ITEM ( 'NONE', ( #36499 ), #40140 ) ;
#36410=DIRECTION ( 'NONE',  ( -4.314083075427411048E-32, -1.000000000000000000, -6.123233995736762338E-17 ) ) ;
#36419=VECTOR ( 'NONE', #56401, 1000.000000000000000 ) ;
#36463=CYLINDRICAL_SURFACE ( 'NONE', #31161, 5.000000000000004441 ) ;
#36499=PRESENTATION_STYLE_ASSIGNMENT (( #25614 ) ) ;
#36511=DIRECTION ( 'NONE',  ( -1.000000000000000000, 0.000000000000000000, -1.337618101958020291E-16 ) ) ;
#36512=SURFACE_SIDE_STYLE ('',( #57628 ) ) ;
#36535=VECTOR ( 'NONE', #6783, 1000.000000000000000 ) ;
#36564=CIRCLE ( 'NONE', #48878, 5.000000000000004441 ) ;
#36586=EDGE_LOOP ( 'NONE', ( #52053, #6853, #9868, #38004 ) ) ;
#36592=( LENGTH_UNIT ( ) NAMED_UNIT ( * ) SI_UNIT ( .MILLI., .METRE. ) );
#36597=LINE ( 'NONE', #9866, #25200 ) ;
#36678=CARTESIAN_POINT ( 'NONE',  ( 447.3372781065083927, 395.0000000000043769, 91.05029585798419589 ) ) ;
#36693=UNCERTAINTY_MEASURE_WITH_UNIT (LENGTH_MEASURE( 1.000000000000000082E-05 ), #37192, 'distance_accuracy_value', 'NONE');
#36710=LINE ( 'NONE', #36356, #54279 ) ;
#36715=ORIENTED_EDGE ( 'NONE', *, *, #50885, .T. ) ;
#36745=CARTESIAN_POINT ( 'NONE',  ( -452.6627218934913230, 177.8591479523843475, -111.4497041420117966 ) ) ;
#36788=ORIENTED_EDGE ( 'NONE', *, *, #69466, .T. ) ;
#36796=VERTEX_POINT ( 'NONE', #48169 ) ;
#36808=VERTEX_POINT ( 'NONE', #43242 ) ;
#36857=ORIENTED_EDGE ( 'NONE', *, *, #5061, .F. ) ;
#36859=ORIENTED_EDGE ( 'NONE', *, *, #28252, .T. ) ;
#36860=PLANE ( 'NONE',  #54227 ) ;
#36863=CARTESIAN_POINT ( 'NONE',  ( -440.1146514826278349, 394.9999999999998295, 101.0022254471246441 ) ) ;
#36866=AXIS2_PLACEMENT_3D ( 'NONE', #699, #69299, #36953 ) ;
#36872=CYLINDRICAL_SURFACE ( 'NONE', #52045, 5.000000000000004441 ) ;
#36878=CARTESIAN_POINT ( 'NONE',  ( -442.6627218934913230, 399.9999999999997726, 108.5502958579881891 ) ) ;
#36880=PLANE ( 'NONE',  #22287 ) ;
#36886=LINE ( 'NONE', #69224, #43556 ) ;
#36893=ORIENTED_EDGE ( 'NONE', *, *, #6501, .T. ) ;
#36912=AXIS2_PLACEMENT_3D ( 'NONE', #46299, #45269, #24529 ) ;
#36914=VERTEX_POINT ( 'NONE', #11945 ) ;
#36937=CARTESIAN_POINT ( 'NONE',  ( 447.3372781065085633, 399.9999999999998863, 78.55029585798817493 ) ) ;
#36942=VERTEX_POINT ( 'NONE', #12299 ) ;
#36953=DIRECTION ( 'NONE',  ( 1.000000000000000000, 0.000000000000000000, 0.000000000000000000 ) ) ;
#36978=ORIENTED_EDGE ( 'NONE', *, *, #50356, .T. ) ;
#36985=ADVANCED_FACE ( 'NONE', ( #28119 ), #17926, .F. ) ;
#36987=CARTESIAN_POINT ( 'NONE',  ( -452.6627218934860934, 395.0000000000064801, -133.9497041420121377 ) ) ;
#36991=EDGE_LOOP ( 'NONE', ( #53141, #25527, #43933, #22855 ) ) ;
#36994=CARTESIAN_POINT ( 'NONE',  ( -452.6627218934912094, 399.9999999999998295, 113.5502958579882602 ) ) ;
#37008=EDGE_CURVE ( 'NONE', #46955, #20487, #16003, .T. ) ;
#37024=ORIENTED_EDGE ( 'NONE', *, *, #55358, .T. ) ;
#37026=CARTESIAN_POINT ( 'NONE',  ( 412.3372781065087906, 400.0000000000065938, -111.4497041420121093 ) ) ;
#37042=DIRECTION ( 'NONE',  ( -1.850371928290090422E-16, 1.000000000000000000, 1.110223024625156171E-16 ) ) ;
#37069=CARTESIAN_POINT ( 'NONE',  ( 437.3372781065091885, 395.0000000000066507, -136.4497041420121661 ) ) ;
#37086=EDGE_CURVE ( 'NONE', #9108, #1887, #16696, .T. ) ;
#37158=DIRECTION ( 'NONE',  ( -1.850169831522831466E-16, 1.000000000000000000, 1.110223024625156294E-16 ) ) ;
#37162=EDGE_CURVE ( 'NONE', #26944, #38916, #6503, .T. ) ;
#37192=( LENGTH_UNIT ( ) NAMED_UNIT ( * ) SI_UNIT ( .MILLI., .METRE. ) );
#37252=ORIENTED_EDGE ( 'NONE', *, *, #54050, .T. ) ;
#37257=PLANE ( 'NONE',  #67127 ) ;
#37261=FACE_OUTER_BOUND ( 'NONE', #50516, .T. ) ;
#37273=DIRECTION ( 'NONE',  ( 1.000000000000000000, 0.000000000000000000, 0.000000000000000000 ) ) ;
#37285=CARTESIAN_POINT ( 'NONE',  ( -422.6627218934914936, 399.9999999999998863, -146.4497041420118251 ) ) ;
#37314=LINE ( 'NONE', #48543, #54732 ) ;
#37326=LINE ( 'NONE', #53499, #7978 ) ;
#37332=CARTESIAN_POINT ( 'NONE',  ( -450.6627218934913230, 177.8591479523843475, -111.4497041420117966 ) ) ;
#37380=ADVANCED_FACE ( 'NONE', ( #34289 ), #66653, .T. ) ;
#37399=VECTOR ( 'NONE', #33749, 1000.000000000000114 ) ;
#37420=AXIS2_PLACEMENT_3D ( 'NONE', #50792, #44828, #18787 ) ;
#37423=ORIENTED_EDGE ( 'NONE', *, *, #23615, .T. ) ;
#37424=LINE ( 'NONE', #4395, #69082 ) ;
#37427=VECTOR ( 'NONE', #44172, 1000.000000000000000 ) ;
#37432=DIRECTION ( 'NONE',  ( -9.109522253334613014E-16, -1.000000000000000000, 3.889846672687432470E-31 ) ) ;
#37441=LINE ( 'NONE', #27585, #12052 ) ;
#37452=ORIENTED_EDGE ( 'NONE', *, *, #3257, .F. ) ;
#37462=EDGE_LOOP ( 'NONE', ( #58240, #17195, #42377, #20538 ) ) ;
#37476=EDGE_CURVE ( 'NONE', #3161, #6104, #5774, .T. ) ;
#37480=ADVANCED_FACE ( 'NONE', ( #63434 ), #10294, .F. ) ;
#37495=CARTESIAN_POINT ( 'NONE',  ( 442.3372781065085633, 392.9289321881414594, -141.4497041420116261 ) ) ;
#37518=DIRECTION ( 'NONE',  ( 1.110223024625156294E-16, 3.697785493223491743E-32, -1.000000000000000000 ) ) ;
#37535=CARTESIAN_POINT ( 'NONE',  ( 1.951563910473907981E-14, 0.000000000000000000, -146.4497041420118251 ) ) ;
#37554=CARTESIAN_POINT ( 'NONE',  ( 299.8372781065085064, 399.9999999999998863, -33.94970414201181796 ) ) ;
#37561=ORIENTED_EDGE ( 'NONE', *, *, #23968, .F. ) ;
#37588=EDGE_LOOP ( 'NONE', ( #50033, #12021, #36857, #67573 ) ) ;
#37592=FACE_OUTER_BOUND ( 'NONE', #66267, .T. ) ;
#37593=DIRECTION ( 'NONE',  ( 8.893845946170152056E-21, -1.110223024625156294E-16, 1.000000000000000000 ) ) ;
#37595=PLANE ( 'NONE',  #39315 ) ;
#37606=LINE ( 'NONE', #5593, #23710 ) ;
#37612=ORIENTED_EDGE ( 'NONE', *, *, #37086, .T. ) ;
#37621=( NAMED_UNIT ( * ) SI_UNIT ( $, .STERADIAN. ) SOLID_ANGLE_UNIT ( ) );
#37636=EDGE_CURVE ( 'NONE', #38916, #22933, #36127, .T. ) ;
#37729=CARTESIAN_POINT ( 'NONE',  ( 442.3372781065086201, 0.000000000000000000, -116.4497041420118393 ) ) ;
#37755=VECTOR ( 'NONE', #11214, 1000.000000000000114 ) ;
#37756=FACE_OUTER_BOUND ( 'NONE', #59068, .T. ) ;
#37758=VERTEX_POINT ( 'NONE', #2532 ) ;
#37761=EDGE_LOOP ( 'NONE', ( #60794, #19595, #58363, #28672 ) ) ;
#37788=ORIENTED_EDGE ( 'NONE', *, *, #38557, .F. ) ;
#37804=DIRECTION ( 'NONE',  ( 1.000000000000000000, 1.850550996349095901E-16, 1.228197773518735191E-20 ) ) ;
#37805=CARTESIAN_POINT ( 'NONE',  ( 437.3372781065086201, 0.000000000000000000, 108.5502958579881749 ) ) ;
#37850=DIRECTION ( 'NONE',  ( -1.850371928290090422E-16, 1.000000000000000000, 1.110223024625156171E-16 ) ) ;
#37856=CARTESIAN_POINT ( 'NONE',  ( 447.3372781065084496, 390.0000000000043769, 108.5502958579838122 ) ) ;
#37860=CIRCLE ( 'NONE', #8662, 5.000000000000004441 ) ;
#37874=ORIENTED_EDGE ( 'NONE', *, *, #47787, .T. ) ;
#37896=PLANE ( 'NONE',  #3038 ) ;
#37907=AXIS2_PLACEMENT_3D ( 'NONE', #33772, #45357, #23565 ) ;
#37920=ORIENTED_EDGE ( 'NONE', *, *, #16884, .F. ) ;
#37922=ORIENTED_EDGE ( 'NONE', *, *, #6501, .F. ) ;
#37924=DIRECTION ( 'NONE',  ( -0.000000000000000000, -6.405132834375902056E-16, 1.000000000000000000 ) ) ;
#37934=EDGE_CURVE ( 'NONE', #8973, #51862, #53461, .T. ) ;
#37943=CARTESIAN_POINT ( 'NONE',  ( 417.3372781065085633, 395.0000000000000568, -116.4497041420117824 ) ) ;
#37946=CARTESIAN_POINT ( 'NONE',  ( 445.3372781065086201, 0.000000000000000000, -1.353084311261909534E-13 ) ) ;
#37947=CARTESIAN_POINT ( 'NONE',  ( 447.3372781065089043, 400.0000000000059117, -146.4497041420121377 ) ) ;
#37962=DIRECTION ( 'NONE',  ( -4.270088556250601699E-16, -0.000000000000000000, -1.000000000000000000 ) ) ;
#37991=ORIENTED_EDGE ( 'NONE', *, *, #28172, .T. ) ;
#37993=FACE_OUTER_BOUND ( 'NONE', #11346, .T. ) ;
#38004=ORIENTED_EDGE ( 'NONE', *, *, #67198, .T. ) ;
#38027=( LENGTH_UNIT ( ) NAMED_UNIT ( * ) SI_UNIT ( .MILLI., .METRE. ) );
#38085=VERTEX_POINT ( 'NONE', #59781 ) ;
#38128=ORIENTED_EDGE ( 'NONE', *, *, #17361, .T. ) ;
#38145=CARTESIAN_POINT ( 'NONE',  ( -443.1918329948323390, 394.9767458440207974, -132.2549152767664964 ) ) ;
#38193=CARTESIAN_POINT ( 'NONE',  ( -452.6627218934915504, 399.9999999999998863, -146.4497041420118251 ) ) ;
#38201=ORIENTED_EDGE ( 'NONE', *, *, #63616, .T. ) ;
#38224=AXIS2_PLACEMENT_3D ( 'NONE', #13570, #62453, #68089 ) ;
#38227=DIRECTION ( 'NONE',  ( -1.850371928290090422E-16, 1.000000000000000000, 1.110223024625156294E-16 ) ) ;
#38249=EDGE_CURVE ( 'NONE', #56564, #38457, #33773, .T. ) ;
#38253=DIRECTION ( 'NONE',  ( 1.000000000000000000, 1.748184826783646563E-16, 0.000000000000000000 ) ) ;
#38266=ORIENTED_EDGE ( 'NONE', *, *, #44386, .T. ) ;
#38275=VECTOR ( 'NONE', #56448, 1000.000000000000000 ) ;
#38286=CARTESIAN_POINT ( 'NONE',  ( -439.4229916354185548, 400.0000000000021032, 91.05029585799266556 ) ) ;
#38314=LINE ( 'NONE', #11229, #67019 ) ;
#38339=CARTESIAN_POINT ( 'NONE',  ( -439.4229916354183842, 388.0000000000064801, -128.9497041420121093 ) ) ;
#38358=CARTESIAN_POINT ( 'NONE',  ( -443.1918329948321684, 394.9767458440207974, 99.35550699274327258 ) ) ;
#38379=DIRECTION ( 'NONE',  ( -1.000000000000000000, 0.000000000000000000, 0.000000000000000000 ) ) ;
#38387=ORIENTED_EDGE ( 'NONE', *, *, #53101, .F. ) ;
#38402=CARTESIAN_POINT ( 'NONE',  ( 442.3372781065085633, 399.9999999999998863, 83.55029585798818914 ) ) ;
#38416=( BOUNDED_CURVE ( )  B_SPLINE_CURVE ( 3, ( #29905, #67893, #14757, #30947 ),
 .UNSPECIFIED., .F., .F. ) 
 B_SPLINE_CURVE_WITH_KNOTS ( ( 4, 4 ),
 ( -8.881784197001252323E-16, 1.570796326794896336 ),
 .UNSPECIFIED. ) 
 CURVE ( )  GEOMETRIC_REPRESENTATION_ITEM ( )  RATIONAL_B_SPLINE_CURVE ( ( 1.000000000000000000, 0.8047378541243649375, 0.8047378541243649375, 1.000000000000000000 ) ) 
 REPRESENTATION_ITEM ( '' )  );
#38417=EDGE_CURVE ( 'NONE', #24527, #36942, #53382, .T. ) ;
#38440=ORIENTED_EDGE ( 'NONE', *, *, #57725, .F. ) ;
#38457=VERTEX_POINT ( 'NONE', #66412 ) ;
#38468=ORIENTED_EDGE ( 'NONE', *, *, #20631, .T. ) ;
#38488=AXIS2_PLACEMENT_3D ( 'NONE', #8899, #19795, #8556 ) ;
#38495=CARTESIAN_POINT ( 'NONE',  ( 112.3013380801408658, 400.0000000000066507, -128.9497041420121093 ) ) ;
#38496=CARTESIAN_POINT ( 'NONE',  ( -452.6627218934915504, 399.9999999999998863, -146.4497041420118251 ) ) ;
#38502=ORIENTED_EDGE ( 'NONE', *, *, #37476, .F. ) ;
#38535=DIRECTION ( 'NONE',  ( -1.020422603260505347E-14, 1.000000000000000000, 5.551115123125782702E-17 ) ) ;
#38552=LINE ( 'NONE', #59997, #66443 ) ;
#38557=EDGE_CURVE ( 'NONE', #67458, #24702, #45970, .T. ) ;
#38561=CARTESIAN_POINT ( 'NONE',  ( 442.3372781065085633, 399.9999999999998863, 103.5502958579881891 ) ) ;
#38595=DIRECTION ( 'NONE',  ( 1.000000000000000000, 1.110223024625155594E-14, -1.110223024625155594E-14 ) ) ;
#38615=CARTESIAN_POINT ( 'NONE',  ( -417.6627218934913230, 179.4906275429376308, -146.4497041420118819 ) ) ;
#38637=VERTEX_POINT ( 'NONE', #62141 ) ;
#38642=FACE_OUTER_BOUND ( 'NONE', #3867, .T. ) ;
#38653=DIRECTION ( 'NONE',  ( 1.697894969632810155E-16, -1.110223024625155801E-16, 1.000000000000000000 ) ) ;
#38665=ORIENTED_EDGE ( 'NONE', *, *, #7644, .T. ) ;
#38693=ORIENTED_EDGE ( 'NONE', *, *, #4757, .F. ) ;
#38702=VERTEX_POINT ( 'NONE', #32551 ) ;
#38715=CARTESIAN_POINT ( 'NONE',  ( -443.6249203811465804, 394.9114286947786354, 98.78386141483146332 ) ) ;
#38721=CARTESIAN_POINT ( 'NONE',  ( -442.6627218934912662, 389.9999999999998295, 113.5502958579881465 ) ) ;
#38734=DIRECTION ( 'NONE',  ( -1.850550996349095901E-16, 1.000000000000000000, -5.551115123125781470E-17 ) ) ;
#38755=DIRECTION ( 'NONE',  ( -0.7071067811865475727, -2.220446049250312341E-16, 0.7071067811865474617 ) ) ;
#38779=ORIENTED_EDGE ( 'NONE', *, *, #1411, .F. ) ;
#38798=CARTESIAN_POINT ( 'NONE',  ( 50.98853755884157835, 388.0000000000065370, -133.9497041420122798 ) ) ;
#38824=ADVANCED_FACE ( 'NONE', ( #7826 ), #40516, .T. ) ;
#38855=UNCERTAINTY_MEASURE_WITH_UNIT (LENGTH_MEASURE( 1.000000000000000082E-05 ), #27409, 'distance_accuracy_value', 'NONE');
#38856=LINE ( 'NONE', #7183, #31524 ) ;
#38880=ORIENTED_EDGE ( 'NONE', *, *, #49509, .F. ) ;
#38898=CARTESIAN_POINT ( 'NONE',  ( 412.3372781065087906, 400.0000000000065938, -111.4497041420121093 ) ) ;
#38916=VERTEX_POINT ( 'NONE', #24701 ) ;
#38977=VECTOR ( 'NONE', #67241, 1000.000000000000000 ) ;
#38998=ORIENTED_EDGE ( 'NONE', *, *, #15515, .F. ) ;
#38999=EDGE_CURVE ( 'NONE', #60543, #11940, #26762, .T. ) ;
#39016=DIRECTION ( 'NONE',  ( -1.020422603260505347E-14, 1.000000000000000000, 5.551115123125782702E-17 ) ) ;
#39062=LINE ( 'NONE', #52377, #67933 ) ;
#39069=FACE_OUTER_BOUND ( 'NONE', #52973, .T. ) ;
#39104=CARTESIAN_POINT ( 'NONE',  ( -444.3843108123961656, 394.6949978562683441, 95.33065306861280419 ) ) ;
#39128=FACE_OUTER_BOUND ( 'NONE', #2464, .T. ) ;
#39178=FACE_OUTER_BOUND ( 'NONE', #59307, .T. ) ;
#39182=ORIENTED_EDGE ( 'NONE', *, *, #68866, .F. ) ;
#39213=CARTESIAN_POINT ( 'NONE',  ( 447.3372781065085633, 399.9999999999998863, 83.55029585798818914 ) ) ;
#39250=VECTOR ( 'NONE', #32403, 1000.000000000000000 ) ;
#39254=CARTESIAN_POINT ( 'NONE',  ( -439.4229916354183842, 400.0000000000065370, -128.9497041420121093 ) ) ;
#39256=( BOUNDED_CURVE ( )  B_SPLINE_CURVE ( 3, ( #3458, #4156, #8396, #25620 ),
 .UNSPECIFIED., .F., .F. ) 
 B_SPLINE_CURVE_WITH_KNOTS ( ( 4, 4 ),
 ( 1.570796326794896558, 3.141592653589793116 ),
 .UNSPECIFIED. ) 
 CURVE ( )  GEOMETRIC_REPRESENTATION_ITEM ( )  RATIONAL_B_SPLINE_CURVE ( ( 1.000000000000000000, 0.8047378541243649375, 0.8047378541243649375, 1.000000000000000000 ) ) 
 REPRESENTATION_ITEM ( '' )  );
#39277=CARTESIAN_POINT ( 'NONE',  ( 442.3372781065085633, 399.9999999999998863, 83.55029585798818914 ) ) ;
#39303=DIRECTION ( 'NONE',  ( 1.000000000000000000, 2.117582368135750246E-20, -1.697742017499683849E-16 ) ) ;
#39315=AXIS2_PLACEMENT_3D ( 'NONE', #37946, #33385, #44258 ) ;
#39320=ORIENTED_EDGE ( 'NONE', *, *, #63368, .F. ) ;
#39353=CARTESIAN_POINT ( 'NONE',  ( -439.4229916354182706, 388.0000000000064233, 91.05029585798840230 ) ) ;
#39359=CARTESIAN_POINT ( 'NONE',  ( 442.3372781065085633, 392.9289321881387878, 108.5502958579838548 ) ) ;
#39432=EDGE_LOOP ( 'NONE', ( #37423, #30262, #64445, #40659 ) ) ;
#39456=ORIENTED_EDGE ( 'NONE', *, *, #12388, .T. ) ;
#39512=FACE_OUTER_BOUND ( 'NONE', #45205, .T. ) ;
#39553=EDGE_CURVE ( 'NONE', #30998, #4775, #51903, .T. ) ;
#39554=EDGE_CURVE ( 'NONE', #22933, #36104, #28537, .T. ) ;
#39577=ADVANCED_FACE ( 'NONE', ( #27478 ), #59484, .F. ) ;
#39588=CARTESIAN_POINT ( 'NONE',  ( 112.3013380801408232, 388.0000000000077307, 101.0502958579874644 ) ) ;
#39602=LINE ( 'NONE', #66359, #39657 ) ;
#39606=AXIS2_PLACEMENT_3D ( 'NONE', #41402, #3759, #62856 ) ;
#39608=CARTESIAN_POINT ( 'NONE',  ( 417.3372781065085633, 400.0000000000000568, -141.4497041420118251 ) ) ;
#39619=PLANE ( 'NONE',  #24079 ) ;
#39642=CYLINDRICAL_SURFACE ( 'NONE', #22245, 4.999999999999990230 ) ;
#39653=EDGE_LOOP ( 'NONE', ( #54132, #35407, #14471, #42482 ) ) ;
#39657=VECTOR ( 'NONE', #23080, 1000.000000000000000 ) ;
#39675=AXIS2_PLACEMENT_3D ( 'NONE', #56854, #19556, #41016 ) ;
#39739=CARTESIAN_POINT ( 'NONE',  ( 437.3372781065085633, 400.0000000000000568, -141.4497041420118251 ) ) ;
#39744=AXIS2_PLACEMENT_3D ( 'NONE', #16496, #27386, #1019 ) ;
#39750=CARTESIAN_POINT ( 'NONE',  ( 447.3372781065085064, 364.9999999999990905, 113.5502958579887007 ) ) ;
#39779=ORIENTED_EDGE ( 'NONE', *, *, #876, .F. ) ;
#39789=EDGE_CURVE ( 'NONE', #3161, #24241, #50679, .T. ) ;
#39822=ORIENTED_EDGE ( 'NONE', *, *, #2955, .T. ) ;
#39827=EDGE_LOOP ( 'NONE', ( #21410, #26054, #18298, #64082 ) ) ;
#39831=VERTEX_POINT ( 'NONE', #20745 ) ;
#39837=ORIENTED_EDGE ( 'NONE', *, *, #49312, .T. ) ;
#39881=ADVANCED_FACE ( 'NONE', ( #22121 ), #16838, .T. ) ;
#39966=LINE ( 'NONE', #29078, #62530 ) ;
#40015=MANIFOLD_SOLID_BREP ( 'Cut-Extrude1[1]', #40655 ) ;
#40025=DIRECTION ( 'NONE',  ( -1.385490305291001461E-14, -1.000000000000000000, -1.110223024625132258E-16 ) ) ;
#40047=SURFACE_STYLE_FILL_AREA ( #34445 ) ;
#40053=CARTESIAN_POINT ( 'NONE',  ( -442.6627218934918915, 395.0000000000064801, -136.4497041420121661 ) ) ;
#40065=ORIENTED_EDGE ( 'NONE', *, *, #40758, .T. ) ;
#40066=DIRECTION ( 'NONE',  ( -1.000000000000000000, -1.001918046209079887E-14, 9.729495617646301779E-15 ) ) ;
#40104=DIRECTION ( 'NONE',  ( -1.000000000000000000, 0.000000000000000000, 0.000000000000000000 ) ) ;
#40131=ORIENTED_EDGE ( 'NONE', *, *, #59715, .T. ) ;
#40138=CARTESIAN_POINT ( 'NONE',  ( 445.3372781065085633, 217.8591479523844612, -111.4497041420119388 ) ) ;
#40140=MANIFOLD_SOLID_BREP ( 'Angle iron 35 X 35 X 5(2)', #45174 ) ;
#40170=AXIS2_PLACEMENT_3D ( 'NONE', #17221, #69311, #58738 ) ;
#40213=CARTESIAN_POINT ( 'NONE',  ( 417.3372781065085633, 400.0000000000000568, -141.4497041420118251 ) ) ;
#40232=CARTESIAN_POINT ( 'NONE',  ( -452.6627218934858661, 400.0000000000064801, -116.4497041420121377 ) ) ;
#40257=DIRECTION ( 'NONE',  ( 0.000000000000000000, 0.000000000000000000, -1.000000000000000000 ) ) ;
#40297=ORIENTED_EDGE ( 'NONE', *, *, #56822, .F. ) ;
#40302=CARTESIAN_POINT ( 'NONE',  ( -452.6627218934859798, 390.0000000000064801, -141.4497041420121377 ) ) ;
#40306=ORIENTED_EDGE ( 'NONE', *, *, #38249, .T. ) ;
#40342=ADVANCED_FACE ( 'NONE', ( #18168 ), #39619, .F. ) ;
#40353=ORIENTED_EDGE ( 'NONE', *, *, #47633, .T. ) ;
#40361=MANIFOLD_SOLID_BREP ( 'Boss-Extrude1', #58612 ) ;
#40372=DIRECTION ( 'NONE',  ( 1.000000000000000000, 1.387778780781442471E-16, 0.000000000000000000 ) ) ;
#40384=ORIENTED_EDGE ( 'NONE', *, *, #24554, .F. ) ;
#40386=ORIENTED_EDGE ( 'NONE', *, *, #46887, .T. ) ;
#40397=DIRECTION ( 'NONE',  ( 9.109522253334654429E-16, 1.000000000000000000, 1.305497313003906699E-14 ) ) ;
#40455=VERTEX_POINT ( 'NONE', #53258 ) ;
#40489=CARTESIAN_POINT ( 'NONE',  ( -439.4229916354184411, 394.9999999999955094, 101.0502958579930066 ) ) ;
#40501=EDGE_CURVE ( 'NONE', #67714, #20392, #12810, .T. ) ;
#40516=CYLINDRICAL_SURFACE ( 'NONE', #25036, 5.000000000000004441 ) ;
#40533=DIRECTION ( 'NONE',  ( -9.109522253334613014E-16, -1.000000000000000000, 3.889846672687432470E-31 ) ) ;
#40549=ORIENTED_EDGE ( 'NONE', *, *, #2948, .F. ) ;
#40579=DIRECTION ( 'NONE',  ( 1.000000000000000000, 1.850550996349095901E-16, 1.228197773518735191E-20 ) ) ;
#40584=ORIENTED_EDGE ( 'NONE', *, *, #1786, .T. ) ;
#40591=CARTESIAN_POINT ( 'NONE',  ( 447.3372781065086201, 370.0000000000043769, 108.5502958579838264 ) ) ;
#40598=VECTOR ( 'NONE', #60986, 1000.000000000000000 ) ;
#40616=PLANE ( 'NONE',  #46618 ) ;
#40631=CARTESIAN_POINT ( 'NONE',  ( 445.3372781065085633, 177.8591479523844612, -111.4497041420119388 ) ) ;
#40655=CLOSED_SHELL ( 'NONE', ( #64072, #19069, #5302, #640, #66941, #34804, #41213, #18844, #17627, #41222, #30966, #24594, #60087, #46222, #58970, #24107, #12303, #48651, #45976, #6971 ) ) ;
#40659=ORIENTED_EDGE ( 'NONE', *, *, #57725, .T. ) ;
#40734=DIRECTION ( 'NONE',  ( -0.000000000000000000, -6.405132834375902056E-16, 1.000000000000000000 ) ) ;
#40739=DIRECTION ( 'NONE',  ( 1.000000000000000000, 1.850550996349095901E-16, 1.228197773518735191E-20 ) ) ;
#40754=VERTEX_POINT ( 'NONE', #37026 ) ;
#40758=EDGE_CURVE ( 'NONE', #33355, #34907, #12637, .T. ) ;
#40793=EDGE_CURVE ( 'NONE', #40754, #48439, #31741, .T. ) ;
#40810=CARTESIAN_POINT ( 'NONE',  ( -450.6627218934913230, 177.8591479523843475, -111.4497041420117966 ) ) ;
#40854=CARTESIAN_POINT ( 'NONE',  ( -452.6627218934914367, 399.9999999999998863, -111.4497041420118251 ) ) ;
#40861=ORIENTED_EDGE ( 'NONE', *, *, #54386, .F. ) ;
#40918=ORIENTED_EDGE ( 'NONE', *, *, #50583, .T. ) ;
#40922=UNCERTAINTY_MEASURE_WITH_UNIT (LENGTH_MEASURE( 1.000000000000000082E-05 ), #46970, 'distance_accuracy_value', 'NONE');
#40935=ORIENTED_EDGE ( 'NONE', *, *, #6798, .T. ) ;
#40936=STYLED_ITEM ( 'NONE', ( #20327 ), #40938 ) ;
#40938=MANIFOLD_SOLID_BREP ( 'Boss-Extrude3', #41763 ) ;
#40947=VECTOR ( 'NONE', #30488, 1000.000000000000000 ) ;
#40958=CARTESIAN_POINT ( 'NONE',  ( -417.6627218934914367, 399.9999999999998863, -146.4497041420118251 ) ) ;
#40973=LINE ( 'NONE', #8970, #13970 ) ;
#40997=PLANE ( 'NONE',  #38224 ) ;
#41002=VERTEX_POINT ( 'NONE', #44562 ) ;
#41016=DIRECTION ( 'NONE',  ( -1.001917834450843231E-14, 1.000000000000000000, -7.216449660063517513E-16 ) ) ;
#41025=DIRECTION ( 'NONE',  ( -1.001915251000354105E-14, 1.000000000000000000, -5.551115123125782702E-17 ) ) ;
#41075=DIRECTION ( 'NONE',  ( 1.387778780781445922E-16, -1.000000000000000000, -3.469446951953615421E-17 ) ) ;
#41109=( BOUNDED_CURVE ( )  B_SPLINE_CURVE ( 3, ( #21182, #9246, #32079, #52153 ),
 .UNSPECIFIED., .F., .F. ) 
 B_SPLINE_CURVE_WITH_KNOTS ( ( 4, 4 ),
 ( 1.570796326794906772, 3.141592653589769135 ),
 .UNSPECIFIED. ) 
 CURVE ( )  GEOMETRIC_REPRESENTATION_ITEM ( )  RATIONAL_B_SPLINE_CURVE ( ( 1.000000000000000000, 0.8047378541243730421, 0.8047378541243730421, 1.000000000000000000 ) ) 
 REPRESENTATION_ITEM ( '' )  );
#41110=VERTEX_POINT ( 'NONE', #34713 ) ;
#41114=DIRECTION ( 'NONE',  ( 1.000000000000000000, 2.263859959510412882E-16, -1.697894969632809662E-16 ) ) ;
#41135=VECTOR ( 'NONE', #53003, 1000.000000000000114 ) ;
#41137=VERTEX_POINT ( 'NONE', #61435 ) ;
#41173=ORIENTED_EDGE ( 'NONE', *, *, #16493, .F. ) ;
#41189=DIRECTION ( 'NONE',  ( -5.333935875449778863E-17, 1.000000000000000000, 6.106226635438359986E-16 ) ) ;
#41213=ADVANCED_FACE ( 'NONE', ( #55815 ), #34012, .T. ) ;
#41221=ORIENTED_EDGE ( 'NONE', *, *, #4654, .F. ) ;
#41222=ADVANCED_FACE ( 'NONE', ( #13933 ), #29086, .T. ) ;
#41255=VERTEX_POINT ( 'NONE', #25880 ) ;
#41266=CARTESIAN_POINT ( 'NONE',  ( -439.4229916354183842, 400.0000000000021032, 101.0502958579930066 ) ) ;
#41312=LINE ( 'NONE', #30070, #33152 ) ;
#41322=DIRECTION ( 'NONE',  ( 1.001917982681609001E-14, -1.000000000000000000, -5.551115123125782702E-17 ) ) ;
#41325=DIRECTION ( 'NONE',  ( -0.000000000000000000, -6.405132834375902056E-16, 1.000000000000000000 ) ) ;
#41327=EDGE_CURVE ( 'NONE', #16476, #20392, #35216, .T. ) ;
#41331=CARTESIAN_POINT ( 'NONE',  ( -452.6627218934913799, 0.000000000000000000, -146.4497041420118251 ) ) ;
#41343=PLANE ( 'NONE',  #27512 ) ;
#41352=ORIENTED_EDGE ( 'NONE', *, *, #17153, .T. ) ;
#41369=DIRECTION ( 'NONE',  ( 1.387778780781446169E-16, -1.000000000000000000, -3.469446951953615421E-17 ) ) ;
#41380=DIRECTION ( 'NONE',  ( 0.000000000000000000, 1.232595164407830672E-32, 1.000000000000000000 ) ) ;
#41398=COLOUR_RGB ( '',0.7921568627450980005, 0.8196078431372548767, 0.9333333333333333481 ) ;
#41402=CARTESIAN_POINT ( 'NONE',  ( 429.8372781065087338, 395.0000000000001137, -128.9497041420121093 ) ) ;
#41405=FACE_OUTER_BOUND ( 'NONE', #24024, .T. ) ;
#41437=PLANE ( 'NONE',  #42239 ) ;
#41441=CARTESIAN_POINT ( 'NONE',  ( 112.3013380801407237, 395.0000000000010800, 96.05029585798746439 ) ) ;
#41465=PLANE ( 'NONE',  #9717 ) ;
#41515=EDGE_LOOP ( 'NONE', ( #61591, #43401, #11844, #9046, #35124 ) ) ;
#41527=VERTEX_POINT ( 'NONE', #63076 ) ;
#41538=VERTEX_POINT ( 'NONE', #53539 ) ;
#41541=SURFACE_SIDE_STYLE ('',( #47151 ) ) ;
#41554=ORIENTED_EDGE ( 'NONE', *, *, #26351, .T. ) ;
#41557=ORIENTED_EDGE ( 'NONE', *, *, #30790, .F. ) ;
#41561=ORIENTED_EDGE ( 'NONE', *, *, #9399, .T. ) ;
#41598=AXIS2_PLACEMENT_3D ( 'NONE', #24489, #50853, #13234 ) ;
#41604=ORIENTED_EDGE ( 'NONE', *, *, #57580, .F. ) ;
#41622=LINE ( 'NONE', #20504, #65708 ) ;
#41683=LINE ( 'NONE', #64167, #20257 ) ;
#41684=FACE_OUTER_BOUND ( 'NONE', #52781, .T. ) ;
#41685=CARTESIAN_POINT ( 'NONE',  ( 412.3372781065085633, 219.4906275429376308, -144.4497041420117682 ) ) ;
#41724=ADVANCED_FACE ( 'NONE', ( #39128 ), #7808, .F. ) ;
#41747=MANIFOLD_SOLID_BREP ( 'Boss-Extrude2', #10318 ) ;
#41763=CLOSED_SHELL ( 'NONE', ( #10210, #21219, #30138, #7741, #47931, #53192 ) ) ;
#41772=EDGE_CURVE ( 'NONE', #3113, #30998, #43118, .T. ) ;
#41791=DIRECTION ( 'NONE',  ( -1.387778780781445676E-16, 1.000000000000000000, 4.294171409582122931E-32 ) ) ;
#41824=CARTESIAN_POINT ( 'NONE',  ( -430.1627218934916073, 400.0000000000064801, 91.05029585798840230 ) ) ;
#41832=DIRECTION ( 'NONE',  ( -0.7071067811865543451, -7.105427357601001070E-15, -0.7071067811865408004 ) ) ;
#41860=DIRECTION ( 'NONE',  ( 0.000000000000000000, -0.000000000000000000, 1.000000000000000000 ) ) ;
#41872=DIRECTION ( 'NONE',  ( -0.7071067811865476838, 6.441404958702661839E-16, -0.7071067811865474617 ) ) ;
#41874=VERTEX_POINT ( 'NONE', #45348 ) ;
#41877=CARTESIAN_POINT ( 'NONE',  ( 444.4083459183744935, 365.0000000000066507, -143.5207719538776132 ) ) ;
#41898=DIRECTION ( 'NONE',  ( 1.000000000000000000, -3.344045254895050726E-17, -0.000000000000000000 ) ) ;
#41904=LINE ( 'NONE', #29973, #66974 ) ;
#41931=CARTESIAN_POINT ( 'NONE',  ( -440.1146514826278349, 400.0000000000064801, 101.0022254471246441 ) ) ;
#41945=LINE ( 'NONE', #9942, #6379 ) ;
#41953=VECTOR ( 'NONE', #62271, 1000.000000000000000 ) ;
#41961=DIRECTION ( 'NONE',  ( -0.7071067811865475727, 4.529112861587823989E-16, -0.7071067811865475727 ) ) ;
#41972=DIRECTION ( 'NONE',  ( 1.000000000000000000, 0.000000000000000000, 0.000000000000000000 ) ) ;
#41998=AXIS2_PLACEMENT_3D ( 'NONE', #1405, #10908, #48868 ) ;
#42038=PLANE ( 'NONE',  #50603 ) ;
#42047=AXIS2_PLACEMENT_3D ( 'NONE', #66895, #12716, #61598 ) ;
#42064=VERTEX_POINT ( 'NONE', #28946 ) ;
#42086=ORIENTED_EDGE ( 'NONE', *, *, #2953, .F. ) ;
#42101=VERTEX_POINT ( 'NONE', #61639 ) ;
#42121=PLANE ( 'NONE',  #35515 ) ;
#42147=CIRCLE ( 'NONE', #11801, 5.000000000000004441 ) ;
#42169=ADVANCED_FACE ( 'NONE', ( #33444 ), #17601, .T. ) ;
#42177=CARTESIAN_POINT ( 'NONE',  ( -439.4229916354182706, 388.0000000000064233, 91.05029585798840230 ) ) ;
#42198=DIRECTION ( 'NONE',  ( -3.081487911019579554E-32, -1.000000000000000000, -3.469446951953612956E-17 ) ) ;
#42202=CARTESIAN_POINT ( 'NONE',  ( 447.3372781065085633, 399.9999999999998863, 113.5502958579881891 ) ) ;
#42208=SURFACE_STYLE_FILL_AREA ( #47128 ) ;
#42220=DIRECTION ( 'NONE',  ( 0.000000000000000000, 1.000000000000000000, 0.000000000000000000 ) ) ;
#42226=DIRECTION ( 'NONE',  ( 1.000000000000000000, 0.000000000000000000, 0.000000000000000000 ) ) ;
#42231=EDGE_CURVE ( 'NONE', #28106, #4215, #28141, .T. ) ;
#42239=AXIS2_PLACEMENT_3D ( 'NONE', #42463, #57617, #9430 ) ;
#42246=ORIENTED_EDGE ( 'NONE', *, *, #53101, .T. ) ;
#42298=DIRECTION ( 'NONE',  ( -1.850371928290090422E-16, 1.000000000000000000, 1.110223024625156171E-16 ) ) ;
#42306=DIRECTION ( 'NONE',  ( -0.7071067811865474617, 0.000000000000000000, 0.7071067811865474617 ) ) ;
#42313=LINE ( 'NONE', #31753, #69036 ) ;
#42327=PLANE ( 'NONE',  #9718 ) ;
#42357=CARTESIAN_POINT ( 'NONE',  ( -439.4229916354182706, 400.0000000000065370, -123.9497041420119530 ) ) ;
#42364=ORIENTED_EDGE ( 'NONE', *, *, #876, .T. ) ;
#42377=ORIENTED_EDGE ( 'NONE', *, *, #49625, .F. ) ;
#42395=FACE_OUTER_BOUND ( 'NONE', #37462, .T. ) ;
#42401=PRODUCT_CONTEXT ( 'NONE', #63726, 'mechanical' ) ;
#42415=CARTESIAN_POINT ( 'NONE',  ( -422.6627218934906978, 394.9999999999998295, 83.55029585798750702 ) ) ;
#42417=CARTESIAN_POINT ( 'NONE',  ( -440.1146514826276075, 394.9999999999998295, -133.9016337311479958 ) ) ;
#42430=CARTESIAN_POINT ( 'NONE',  ( 442.3372781065085633, 399.9999999999998863, 103.5502958579881891 ) ) ;
#42452=DIRECTION ( 'NONE',  ( 1.387778780781445429E-16, -1.000000000000000000, -3.081487911019577365E-33 ) ) ;
#42458=EDGE_CURVE ( 'NONE', #12369, #58185, #55491, .T. ) ;
#42463=CARTESIAN_POINT ( 'NONE',  ( 412.3372781065085633, 219.4906275429376308, 111.5502958579881749 ) ) ;
#42482=ORIENTED_EDGE ( 'NONE', *, *, #58661, .T. ) ;
#42508=( GEOMETRIC_REPRESENTATION_CONTEXT ( 3 ) GLOBAL_UNCERTAINTY_ASSIGNED_CONTEXT ( ( #51489 ) ) GLOBAL_UNIT_ASSIGNED_CONTEXT ( ( #8038, #3122, #56221 ) ) REPRESENTATION_CONTEXT ( 'NONE', 'WORKASPACE' ) );
#42533=DIRECTION ( 'NONE',  ( -1.000000000000000000, 1.232595164407830946E-32, 7.703719777548943412E-34 ) ) ;
#42540=EDGE_CURVE ( 'NONE', #4404, #68395, #48040, .T. ) ;
#42554=VERTEX_POINT ( 'NONE', #57237 ) ;
#42576=ORIENTED_EDGE ( 'NONE', *, *, #1786, .F. ) ;
#42586=EDGE_CURVE ( 'NONE', #10801, #29739, #26942, .T. ) ;
#42611=CARTESIAN_POINT ( 'NONE',  ( 429.8372781065087906, 400.0000000000067075, -128.9497041420121093 ) ) ;
#42615=CARTESIAN_POINT ( 'NONE',  ( -452.6627218934914936, 364.9999999999953957, 113.5502958579925945 ) ) ;
#42674=ORIENTED_EDGE ( 'NONE', *, *, #14132, .T. ) ;
#42707=LINE ( 'NONE', #20222, #1242 ) ;
#42712=CARTESIAN_POINT ( 'NONE',  ( -439.4229916354183842, 394.9999999999998295, -128.9497041420121093 ) ) ;
#42773=EDGE_CURVE ( 'NONE', #45699, #68395, #40973, .T. ) ;
#42825=VERTEX_POINT ( 'NONE', #62780 ) ;
#42832=ORIENTED_EDGE ( 'NONE', *, *, #42586, .F. ) ;
#42860=FACE_OUTER_BOUND ( 'NONE', #33827, .T. ) ;
#42935=EDGE_CURVE ( 'NONE', #26400, #6906, #12930, .T. ) ;
#42953=EDGE_LOOP ( 'NONE', ( #44769, #68209, #54473, #33996 ) ) ;
#42973=CARTESIAN_POINT ( 'NONE',  ( 447.3372781065086201, 177.8591479523844612, 78.55029585798806124 ) ) ;
#42981=CARTESIAN_POINT ( 'NONE',  ( -430.1627218934915504, 400.0000000000065370, -123.9497041420119530 ) ) ;
#42982=DIRECTION ( 'NONE',  ( 0.7071067811865477948, -9.875400524329059797E-15, 0.7071067811865473507 ) ) ;
#43037=AXIS2_PLACEMENT_3D ( 'NONE', #29011, #29340, #66643 ) ;
#43047=LINE ( 'NONE', #23001, #68562 ) ;
#43053=ORIENTED_EDGE ( 'NONE', *, *, #41772, .F. ) ;
#43073=DIRECTION ( 'NONE',  ( 1.000000000000000000, 0.000000000000000000, 1.337618101958020291E-16 ) ) ;
#43118=CIRCLE ( 'NONE', #31889, 5.000000000000170530 ) ;
#43136=AXIS2_PLACEMENT_3D ( 'NONE', #38339, #33432, #12313 ) ;
#43149=DIRECTION ( 'NONE',  ( -9.109522253334613014E-16, -1.000000000000000000, 3.889846672687432470E-31 ) ) ;
#43151=PLANE ( 'NONE',  #47456 ) ;
#43189=ORIENTED_EDGE ( 'NONE', *, *, #44417, .T. ) ;
#43203=( NAMED_UNIT ( * ) PLANE_ANGLE_UNIT ( ) SI_UNIT ( $, .RADIAN. ) );
#43213=DIRECTION ( 'NONE',  ( 1.000000000000000000, 0.000000000000000000, -1.697894969632810155E-16 ) ) ;
#43215=CARTESIAN_POINT ( 'NONE',  ( -417.6627218934913230, 399.9999999999998295, 113.5502958579882602 ) ) ;
#43220=CARTESIAN_POINT ( 'NONE',  ( 447.3372781065085064, 365.0000000000043769, 113.5502958579838122 ) ) ;
#43229=ORIENTED_EDGE ( 'NONE', *, *, #15435, .T. ) ;
#43230=CARTESIAN_POINT ( 'NONE',  ( -439.4229916354184979, 388.0000000000064801, -128.9497041420121093 ) ) ;
#43234=CARTESIAN_POINT ( 'NONE',  ( 112.3013380801408658, 400.0000000000066507, -133.9497041420121377 ) ) ;
#43240=ORIENTED_EDGE ( 'NONE', *, *, #20232, .F. ) ;
#43242=CARTESIAN_POINT ( 'NONE',  ( -439.4229916354184979, 400.0000000000065370, -133.9497041420121377 ) ) ;
#43246=CARTESIAN_POINT ( 'NONE',  ( 437.3372781065085633, 394.9999999999999432, 103.5502958579882460 ) ) ;
#43247=DIRECTION ( 'NONE',  ( 1.940875045995544638E-32, -1.110223024625156171E-16, 1.000000000000000000 ) ) ;
#43263=CIRCLE ( 'NONE', #10745, 5.000000000000004441 ) ;
#43283=LINE ( 'NONE', #12340, #10753 ) ;
#43310=EDGE_CURVE ( 'NONE', #48257, #55132, #43463, .T. ) ;
#43314=ORIENTED_EDGE ( 'NONE', *, *, #37008, .T. ) ;
#43331=CARTESIAN_POINT ( 'NONE',  ( -442.6627218934912662, 394.9999999999998295, 113.5502958579882034 ) ) ;
#43343=CARTESIAN_POINT ( 'NONE',  ( -440.1146514826278349, 400.0000000000021032, 101.0022254471289358 ) ) ;
#43351=ORIENTED_EDGE ( 'NONE', *, *, #58508, .T. ) ;
#43356=ORIENTED_EDGE ( 'NONE', *, *, #23118, .F. ) ;
#43359=EDGE_CURVE ( 'NONE', #41874, #26400, #68415, .T. ) ;
#43401=ORIENTED_EDGE ( 'NONE', *, *, #67988, .T. ) ;
#43415=DIRECTION ( 'NONE',  ( 1.387778780781445922E-16, -1.000000000000000000, -1.232595164407830946E-32 ) ) ;
#43430=ORIENTED_EDGE ( 'NONE', *, *, #1666, .F. ) ;
#43458=VECTOR ( 'NONE', #4515, 1000.000000000000000 ) ;
#43463=LINE ( 'NONE', #11114, #24124 ) ;
#43466=DIRECTION ( 'NONE',  ( 1.000000000000000000, 2.465190328815660250E-32, 0.000000000000000000 ) ) ;
#43496=CARTESIAN_POINT ( 'NONE',  ( 429.8372781065087338, 400.0000000000067075, -128.9497041420121093 ) ) ;
#43498=CARTESIAN_POINT ( 'NONE',  ( -450.6627218934913230, 177.8591479523843475, 78.55029585798814651 ) ) ;
#43547=ORIENTED_EDGE ( 'NONE', *, *, #42773, .F. ) ;
#43554=SURFACE_SIDE_STYLE ('',( #69263 ) ) ;
#43556=VECTOR ( 'NONE', #21053, 1000.000000000000000 ) ;
#43564=ORIENTED_EDGE ( 'NONE', *, *, #53399, .F. ) ;
#43571=AXIS2_PLACEMENT_3D ( 'NONE', #53966, #27250, #48685 ) ;
#43575=CARTESIAN_POINT ( 'NONE',  ( -442.6627218934912662, 394.9999999999998295, 113.5502958579881465 ) ) ;
#43591=EDGE_CURVE ( 'NONE', #53656, #66593, #18405, .T. ) ;
#43609=CARTESIAN_POINT ( 'NONE',  ( -430.1627218934916073, 400.0000000000065370, -123.9497041420119530 ) ) ;
#43624=VERTEX_POINT ( 'NONE', #7159 ) ;
#43634=VERTEX_POINT ( 'NONE', #40213 ) ;
#43651=DIRECTION ( 'NONE',  ( -1.020422603260505347E-14, 1.000000000000000000, 5.551115123125782702E-17 ) ) ;
#43655=EDGE_CURVE ( 'NONE', #57073, #16392, #29653, .T. ) ;
#43678=DIRECTION ( 'NONE',  ( 1.387778780781445429E-16, -1.000000000000000000, -3.081487911019577365E-33 ) ) ;
#43695=DIRECTION ( 'NONE',  ( 0.000000000000000000, 1.232595164407830672E-32, -1.000000000000000000 ) ) ;
#43715=ORIENTED_EDGE ( 'NONE', *, *, #30439, .T. ) ;
#43716=VECTOR ( 'NONE', #45180, 1000.000000000000000 ) ;
#43720=DIRECTION ( 'NONE',  ( 1.000000000000000000, -3.344045254895050726E-17, 0.000000000000000000 ) ) ;
#43744=( BOUNDED_CURVE ( )  B_SPLINE_CURVE ( 3, ( #320, #26723, #30709, #43220 ),
 .UNSPECIFIED., .F., .F. ) 
 B_SPLINE_CURVE_WITH_KNOTS ( ( 4, 4 ),
 ( -8.881784197001252323E-16, 1.570796326794900111 ),
 .UNSPECIFIED. ) 
 CURVE ( )  GEOMETRIC_REPRESENTATION_ITEM ( )  RATIONAL_B_SPLINE_CURVE ( ( 1.000000000000000000, 0.8047378541243640493, 0.8047378541243640493, 1.000000000000000000 ) ) 
 REPRESENTATION_ITEM ( '' )  );
#43837=EDGE_CURVE ( 'NONE', #32464, #22995, #36564, .T. ) ;
#43855=FACE_OUTER_BOUND ( 'NONE', #42953, .T. ) ;
#43861=FACE_OUTER_BOUND ( 'NONE', #48584, .T. ) ;
#43879=ORIENTED_EDGE ( 'NONE', *, *, #44800, .T. ) ;
#43905=DIRECTION ( 'NONE',  ( -6.405487610868040568E-16, -1.000000000000000000, 5.551115123125781470E-17 ) ) ;
#43914=FILL_AREA_STYLE ('',( #54464 ) ) ;
#43920=PLANE ( 'NONE',  #27422 ) ;
#43929=FILL_AREA_STYLE ('',( #65059 ) ) ;
#43932=VECTOR ( 'NONE', #19920, 1000.000000000000000 ) ;
#43933=ORIENTED_EDGE ( 'NONE', *, *, #42231, .T. ) ;
#43950=CARTESIAN_POINT ( 'NONE',  ( 437.3372781065085633, 394.9999999999999432, 103.5502958579882460 ) ) ;
#43957=EDGE_CURVE ( 'NONE', #17566, #16392, #41312, .T. ) ;
#43968=ORIENTED_EDGE ( 'NONE', *, *, #49435, .T. ) ;
#43976=ADVANCED_FACE ( 'NONE', ( #61717 ), #19497, .T. ) ;
#43986=FILL_AREA_STYLE_COLOUR ( '', #18949 ) ;
#44002=CARTESIAN_POINT ( 'NONE',  ( -444.4229916354184979, 394.6798985497181320, 96.05029585798874336 ) ) ;
#44024=LINE ( 'NONE', #1133, #67777 ) ;
#44071=FACE_OUTER_BOUND ( 'NONE', #49465, .T. ) ;
#44079=ORIENTED_EDGE ( 'NONE', *, *, #14468, .T. ) ;
#44083=CARTESIAN_POINT ( 'NONE',  ( 447.3372781065086201, 0.000000000000000000, -1.318389841742373392E-13 ) ) ;
#44125=VECTOR ( 'NONE', #34100, 1000.000000000000000 ) ;
#44132=AXIS2_PLACEMENT_3D ( 'NONE', #16924, #65839, #49273 ) ;
#44135=CARTESIAN_POINT ( 'NONE',  ( 447.3372781065087338, 365.0000000000043769, 113.5502958579838122 ) ) ;
#44136=AXIS2_PLACEMENT_3D ( 'NONE', #24903, #46334, #67811 ) ;
#44145=CARTESIAN_POINT ( 'NONE',  ( 417.3372781065091317, 395.0000000000065938, -116.4497041420121661 ) ) ;
#44155=FACE_OUTER_BOUND ( 'NONE', #59051, .T. ) ;
#44172=DIRECTION ( 'NONE',  ( -1.850169831522831466E-16, 1.000000000000000000, 1.110223024625156294E-16 ) ) ;
#44187=DIRECTION ( 'NONE',  ( 1.387778780781445429E-16, -1.000000000000000000, -3.081487911019577365E-33 ) ) ;
#44226=EDGE_LOOP ( 'NONE', ( #49016, #7621, #50888, #16718, #829, #66280, #11671, #55237, #66824, #23739 ) ) ;
#44256=CARTESIAN_POINT ( 'NONE',  ( 429.8372781065087338, 400.0000000000067075, -133.9497041420121377 ) ) ;
#44258=DIRECTION ( 'NONE',  ( -2.921639538487254261E-16, -1.134144525784205431E-35, -1.000000000000000000 ) ) ;
#44274=DIRECTION ( 'NONE',  ( 0.7071067811865476838, -6.441404958702661839E-16, 0.7071067811865474617 ) ) ;
#44295=VECTOR ( 'NONE', #44274, 1000.000000000000000 ) ;
#44344=CARTESIAN_POINT ( 'NONE',  ( -452.6627218934859798, 400.0000000000064801, -111.4497041420121661 ) ) ;
#44386=EDGE_CURVE ( 'NONE', #42554, #42825, #20041, .T. ) ;
#44388=ADVANCED_FACE ( 'NONE', ( #56279 ), #36215, .T. ) ;
#44417=EDGE_CURVE ( 'NONE', #51074, #68125, #30943, .T. ) ;
#44460=VECTOR ( 'NONE', #53846, 1000.000000000000000 ) ;
#44523=CARTESIAN_POINT ( 'NONE',  ( 442.3372781065085633, 399.9999999999998863, 103.5502958579881891 ) ) ;
#44558=DIRECTION ( 'NONE',  ( 0.000000000000000000, 0.000000000000000000, 1.000000000000000000 ) ) ;
#44559=ORIENTED_EDGE ( 'NONE', *, *, #49435, .F. ) ;
#44562=CARTESIAN_POINT ( 'NONE',  ( -447.6627218934914367, 399.9999999999998863, -136.4497041420118251 ) ) ;
#44603=ADVANCED_FACE ( 'NONE', ( #44155 ), #47437, .T. ) ;
#44619=EDGE_CURVE ( 'NONE', #3113, #11742, #15454, .T. ) ;
#44631=DIRECTION ( 'NONE',  ( 0.000000000000000000, 0.000000000000000000, 1.000000000000000000 ) ) ;
#44644=DIRECTION ( 'NONE',  ( -5.295264586242884027E-16, -1.000000000000000000, -1.110223024625156294E-16 ) ) ;
#44657=EDGE_CURVE ( 'NONE', #22785, #1784, #18141, .T. ) ;
#44677=ORIENTED_EDGE ( 'NONE', *, *, #27366, .F. ) ;
#44699=DIRECTION ( 'NONE',  ( 1.387778780781445922E-16, -1.000000000000000000, -1.232595164407830946E-32 ) ) ;
#44714=EDGE_CURVE ( 'NONE', #68321, #12229, #45546, .T. ) ;
#44719=CARTESIAN_POINT ( 'NONE',  ( -439.4229916354183274, 388.0000000000020464, 101.0502958579930066 ) ) ;
#44769=ORIENTED_EDGE ( 'NONE', *, *, #6435, .T. ) ;
#44799=ORIENTED_EDGE ( 'NONE', *, *, #15811, .F. ) ;
#44800=EDGE_CURVE ( 'NONE', #13434, #13335, #12872, .T. ) ;
#44823=CARTESIAN_POINT ( 'NONE',  ( 1.951563910473907981E-14, 0.000000000000000000, -144.4497041420118251 ) ) ;
#44828=DIRECTION ( 'NONE',  ( 0.7071067811865474617, 0.000000000000000000, -0.7071067811865476838 ) ) ;
#44830=EDGE_CURVE ( 'NONE', #63892, #64521, #61733, .T. ) ;
#44845=ORIENTED_EDGE ( 'NONE', *, *, #54386, .T. ) ;
#44959=FILL_AREA_STYLE_COLOUR ( '', #41398 ) ;
#44967=VERTEX_POINT ( 'NONE', #10338 ) ;
#44977=CARTESIAN_POINT ( 'NONE',  ( 440.2662102946430309, 395.0000000000043769, 106.4792280461184077 ) ) ;
#44978=CARTESIAN_POINT ( 'NONE',  ( 442.3372781065085633, 390.0000000000001137, 108.5502958579883170 ) ) ;
#44995=DIRECTION ( 'NONE',  ( -3.038581678643134250E-64, 1.232595164407830672E-32, 1.000000000000000000 ) ) ;
#45047=LINE ( 'NONE', #55251, #46724 ) ;
#45073=ORIENTED_EDGE ( 'NONE', *, *, #59385, .F. ) ;
#45174=CLOSED_SHELL ( 'NONE', ( #39577, #60253, #60803, #52335, #12584, #43976, #35667, #24699, #14385 ) ) ;
#45180=DIRECTION ( 'NONE',  ( 1.387778780781445922E-16, -1.000000000000000000, -1.232595164407830946E-32 ) ) ;
#45183=ORIENTED_EDGE ( 'NONE', *, *, #66153, .F. ) ;
#45195=DIRECTION ( 'NONE',  ( -4.270088556250601699E-16, -0.000000000000000000, -1.000000000000000000 ) ) ;
#45205=EDGE_LOOP ( 'NONE', ( #69426, #23870, #52984, #29245, #59169 ) ) ;
#45213=EDGE_CURVE ( 'NONE', #24336, #63892, #35625, .T. ) ;
#45246=DIRECTION ( 'NONE',  ( 1.001915251000354105E-14, -1.000000000000000000, -5.551115123135531297E-17 ) ) ;
#45261=ORIENTED_EDGE ( 'NONE', *, *, #41327, .F. ) ;
#45269=DIRECTION ( 'NONE',  ( 1.850169831522831466E-16, -1.000000000000000000, 5.551115123125781470E-17 ) ) ;
#45317=( LENGTH_UNIT ( ) NAMED_UNIT ( * ) SI_UNIT ( .MILLI., .METRE. ) );
#45343=EDGE_CURVE ( 'NONE', #51074, #40455, #29997, .T. ) ;
#45345=ORIENTED_EDGE ( 'NONE', *, *, #57580, .T. ) ;
#45348=CARTESIAN_POINT ( 'NONE',  ( -417.6627218934913230, 399.9999999999997726, 113.5502958579881891 ) ) ;
#45357=DIRECTION ( 'NONE',  ( 4.314083075427411048E-32, 1.000000000000000000, 6.123233995736763571E-17 ) ) ;
#45362=VECTOR ( 'NONE', #41189, 1000.000000000000000 ) ;
#45368=VERTEX_POINT ( 'NONE', #59819 ) ;
#45369=CARTESIAN_POINT ( 'NONE',  ( -452.6627218934912662, 364.9999999999998863, 113.5502958579877912 ) ) ;
#45378=ORIENTED_EDGE ( 'NONE', *, *, #15811, .T. ) ;
#45381=DIRECTION ( 'NONE',  ( -0.7071067811865543451, -7.105427357601001070E-15, -0.7071067811865408004 ) ) ;
#45396=PLANE ( 'NONE',  #8992 ) ;
#45402=LINE ( 'NONE', #24656, #27323 ) ;
#45406=( GEOMETRIC_REPRESENTATION_CONTEXT ( 3 ) GLOBAL_UNCERTAINTY_ASSIGNED_CONTEXT ( ( #40922 ) ) GLOBAL_UNIT_ASSIGNED_CONTEXT ( ( #46970, #15649, #20570 ) ) REPRESENTATION_CONTEXT ( 'NONE', 'WORKASPACE' ) );
#45412=PLANE ( 'NONE',  #42047 ) ;
#45419=CARTESIAN_POINT ( 'NONE',  ( 447.3372781065085633, 400.0000000000000568, -146.4497041420117966 ) ) ;
#45427=DIRECTION ( 'NONE',  ( -1.334402673828311663E-15, 1.000000000000000000, -1.465981474576325310E-14 ) ) ;
#45445=ORIENTED_EDGE ( 'NONE', *, *, #7644, .F. ) ;
#45466=PLANE ( 'NONE',  #1788 ) ;
#45481=EDGE_LOOP ( 'NONE', ( #52131, #15056, #47614, #54261 ) ) ;
#45504=DIRECTION ( 'NONE',  ( 1.850371928290090422E-16, -1.000000000000000000, -1.110223024625156294E-16 ) ) ;
#45517=VECTOR ( 'NONE', #7590, 1000.000000000000000 ) ;
#45519=CYLINDRICAL_SURFACE ( 'NONE', #32761, 5.000000000000004441 ) ;
#45528=ORIENTED_EDGE ( 'NONE', *, *, #1411, .T. ) ;
#45546=CIRCLE ( 'NONE', #48933, 5.000000000000060396 ) ;
#45571=DIRECTION ( 'NONE',  ( -1.850169831522831466E-16, 1.000000000000000000, 1.110223024625156294E-16 ) ) ;
#45598=DIRECTION ( 'NONE',  ( 0.000000000000000000, -6.123233995736762338E-17, 1.000000000000000000 ) ) ;
#45606=CIRCLE ( 'NONE', #56863, 5.000000000000004441 ) ;
#45618=EDGE_CURVE ( 'NONE', #9937, #31046, #46779, .T. ) ;
#45676=ORIENTED_EDGE ( 'NONE', *, *, #20546, .T. ) ;
#45678=CARTESIAN_POINT ( 'NONE',  ( -449.7337897053572533, 365.0000000000064233, -143.5207719538776132 ) ) ;
#45699=VERTEX_POINT ( 'NONE', #37943 ) ;
#45719=EDGE_LOOP ( 'NONE', ( #68129, #22864, #54055, #59549, #20262, #38201, #46497, #17862, #45261, #40861, #13432, #1981, #58284, #38387, #24543 ) ) ;
#45742=ADVANCED_FACE ( 'NONE', ( #42860 ), #64330, .F. ) ;
#45773=CARTESIAN_POINT ( 'NONE',  ( 442.3372781065089612, 370.0000000000065938, -141.4497041420121661 ) ) ;
#45803=DIRECTION ( 'NONE',  ( 1.000000000000000000, -1.604841615724182364E-15, -4.270088556250601699E-16 ) ) ;
#45813=AXIS2_PLACEMENT_3D ( 'NONE', #35271, #8546, #20127 ) ;
#45834=DIRECTION ( 'NONE',  ( 1.000000000000000000, 0.000000000000000000, -7.703719777548943412E-34 ) ) ;
#45852=FACE_OUTER_BOUND ( 'NONE', #8838, .T. ) ;
#45856=UNCERTAINTY_MEASURE_WITH_UNIT (LENGTH_MEASURE( 1.000000000000000082E-05 ), #67079, 'distance_accuracy_value', 'NONE');
#45860=DIRECTION ( 'NONE',  ( 0.000000000000000000, -3.697785493223491743E-32, 1.000000000000000000 ) ) ;
#45861=DIRECTION ( 'NONE',  ( -1.387778780781445922E-16, 1.000000000000000000, 1.232595164407830946E-32 ) ) ;
#45879=VERTEX_POINT ( 'NONE', #44256 ) ;
#45909=ORIENTED_EDGE ( 'NONE', *, *, #24838, .F. ) ;
#45913=DIRECTION ( 'NONE',  ( 1.387778780781445429E-16, -1.000000000000000000, -3.081487911019577365E-33 ) ) ;
#45914=LINE ( 'NONE', #56825, #55656 ) ;
#45961=ADVANCED_FACE ( 'NONE', ( #2752 ), #18929, .F. ) ;
#45970=LINE ( 'NONE', #57222, #67668 ) ;
#45976=ADVANCED_FACE ( 'NONE', ( #35803 ), #35100, .F. ) ;
#45988=ORIENTED_EDGE ( 'NONE', *, *, #59678, .T. ) ;
#46004=EDGE_CURVE ( 'NONE', #22806, #9149, #4811, .T. ) ;
#46015=CARTESIAN_POINT ( 'NONE',  ( 112.3013380801407237, 395.0000000000010800, 96.05029585798746439 ) ) ;
#46079=VECTOR ( 'NONE', #13571, 1000.000000000000000 ) ;
#46082=( NAMED_UNIT ( * ) SI_UNIT ( $, .STERADIAN. ) SOLID_ANGLE_UNIT ( ) );
#46109=DIRECTION ( 'NONE',  ( 1.000000000000000000, 1.387778780781445676E-16, -1.110223024625156294E-16 ) ) ;
#46136=DIRECTION ( 'NONE',  ( -0.000000000000000000, -6.405132834375902056E-16, 1.000000000000000000 ) ) ;
#46151=CARTESIAN_POINT ( 'NONE',  ( -443.1884682831975510, 394.9771332441898721, -125.6405780647352231 ) ) ;
#46157=ORIENTED_EDGE ( 'NONE', *, *, #12499, .T. ) ;
#46178=AXIS2_PLACEMENT_3D ( 'NONE', #36994, #68326, #25070 ) ;
#46185=ORIENTED_EDGE ( 'NONE', *, *, #55358, .F. ) ;
#46198=DIRECTION ( 'NONE',  ( -0.000000000000000000, 1.000000000000000000, -0.000000000000000000 ) ) ;
#46222=ADVANCED_FACE ( 'NONE', ( #68343 ), #69008, .T. ) ;
#46229=LINE ( 'NONE', #64482, #59534 ) ;
#46238=VERTEX_POINT ( 'NONE', #7612 ) ;
#46260=FACE_OUTER_BOUND ( 'NONE', #58874, .T. ) ;
#46261=CARTESIAN_POINT ( 'NONE',  ( -452.6627218934913799, 400.0000000000079581, 113.5502958579925803 ) ) ;
#46283=CARTESIAN_POINT ( 'NONE',  ( -447.6627218934913799, 389.9999999999998295, -141.4497041420118535 ) ) ;
#46299=CARTESIAN_POINT ( 'NONE',  ( 112.3013380801408800, 395.0000000000065938, -128.9497041420121093 ) ) ;
#46307=EDGE_CURVE ( 'NONE', #68321, #4215, #41945, .T. ) ;
#46322=AXIS2_PLACEMENT_3D ( 'NONE', #50399, #27894, #1160 ) ;
#46334=DIRECTION ( 'NONE',  ( 1.000000000000000000, 0.000000000000000000, 1.110223024625156294E-16 ) ) ;
#46353=CARTESIAN_POINT ( 'NONE',  ( -417.6627218934913230, 219.4906275429376308, 111.5502958579881749 ) ) ;
#46383=LINE ( 'NONE', #67862, #18058 ) ;
#46394=ORIENTED_EDGE ( 'NONE', *, *, #8526, .T. ) ;
#46462=( NAMED_UNIT ( * ) SI_UNIT ( $, .STERADIAN. ) SOLID_ANGLE_UNIT ( ) );
#46473=EDGE_CURVE ( 'NONE', #8003, #41002, #66201, .T. ) ;
#46492=COLOUR_RGB ( '',0.7921568627450980005, 0.8196078431372548767, 0.9333333333333333481 ) ;
#46497=ORIENTED_EDGE ( 'NONE', *, *, #40793, .T. ) ;
#46499=PRODUCT_DEFINITION ( 'UNKNOWN', '', #48996, #64099 ) ;
#46500=ORIENTED_EDGE ( 'NONE', *, *, #29645, .T. ) ;
#46507=VECTOR ( 'NONE', #3892, 1000.000000000000000 ) ;
#46524=AXIS2_PLACEMENT_3D ( 'NONE', #49030, #16691, #37804 ) ;
#46529=DIRECTION ( 'NONE',  ( 1.110223024625156294E-16, 3.697785493223491743E-32, -1.000000000000000000 ) ) ;
#46549=VECTOR ( 'NONE', #47694, 1000.000000000000000 ) ;
#46556=CARTESIAN_POINT ( 'NONE',  ( 112.3013380801408658, 388.0000000000065370, 91.05029585798857283 ) ) ;
#46570=ORIENTED_EDGE ( 'NONE', *, *, #29371, .F. ) ;
#46583=LINE ( 'NONE', #24113, #18612 ) ;
#46609=AXIS2_PLACEMENT_3D ( 'NONE', #11063, #69461, #26217 ) ;
#46616=VECTOR ( 'NONE', #64485, 1000.000000000000000 ) ;
#46618=AXIS2_PLACEMENT_3D ( 'NONE', #57155, #30415, #41322 ) ;
#46665=AXIS2_PLACEMENT_3D ( 'NONE', #35006, #35353, #19511 ) ;
#46676=ORIENTED_EDGE ( 'NONE', *, *, #9399, .F. ) ;
#46683=VERTEX_POINT ( 'NONE', #35901 ) ;
#46693=LINE ( 'NONE', #19977, #63199 ) ;
#46703=EDGE_CURVE ( 'NONE', #30998, #68286, #5935, .T. ) ;
#46719=CARTESIAN_POINT ( 'NONE',  ( 412.3372781065086201, 400.0000000000000568, -146.4497041420118251 ) ) ;
#46724=VECTOR ( 'NONE', #65832, 1000.000000000000000 ) ;
#46731=VERTEX_POINT ( 'NONE', #21432 ) ;
#46779=LINE ( 'NONE', #2838, #26513 ) ;
#46784=ORIENTED_EDGE ( 'NONE', *, *, #2884, .F. ) ;
#46791=CARTESIAN_POINT ( 'NONE',  ( 429.8372781065087338, 400.0000000000066507, 96.05029585798857283 ) ) ;
#46807=CARTESIAN_POINT ( 'NONE',  ( -417.6627218934917778, 400.0000000000064801, -111.4497041420121661 ) ) ;
#46815=( LENGTH_UNIT ( ) NAMED_UNIT ( * ) SI_UNIT ( .MILLI., .METRE. ) );
#46826=DIRECTION ( 'NONE',  ( 1.020422603260505347E-14, -1.000000000000000000, -5.551115123125782702E-17 ) ) ;
#46848=CARTESIAN_POINT ( 'NONE',  ( 442.3372781065084496, 390.0000000000043201, 108.5502958579838690 ) ) ;
#46850=EDGE_CURVE ( 'NONE', #6017, #61415, #67156, .T. ) ;
#46862=CIRCLE ( 'NONE', #5286, 5.000000000000004441 ) ;
#46878=CARTESIAN_POINT ( 'NONE',  ( -422.6627218934913230, 399.9999999999997726, 108.5502958579881891 ) ) ;
#46887=EDGE_CURVE ( 'NONE', #34711, #57676, #58092, .T. ) ;
#46890=VERTEX_POINT ( 'NONE', #9432 ) ;
#46924=VERTEX_POINT ( 'NONE', #50955 ) ;
#46940=LINE ( 'NONE', #50833, #2891 ) ;
#46955=VERTEX_POINT ( 'NONE', #69194 ) ;
#46970=( LENGTH_UNIT ( ) NAMED_UNIT ( * ) SI_UNIT ( .MILLI., .METRE. ) );
#46989=LINE ( 'NONE', #3394, #61278 ) ;
#47031=DIRECTION ( 'NONE',  ( 0.000000000000000000, 0.000000000000000000, -1.000000000000000000 ) ) ;
#47034=ORIENTED_EDGE ( 'NONE', *, *, #43837, .F. ) ;
#47038=DIRECTION ( 'NONE',  ( -0.000000000000000000, -6.405132834375902056E-16, 1.000000000000000000 ) ) ;
#47042=CARTESIAN_POINT ( 'NONE',  ( -450.6627218934913230, 0.000000000000000000, -6.938893903907228378E-15 ) ) ;
#47128=FILL_AREA_STYLE ('',( #15130 ) ) ;
#47146=AXIS2_PLACEMENT_3D ( 'NONE', #6247, #63359, #68296 ) ;
#47151=SURFACE_STYLE_FILL_AREA ( #51416 ) ;
#47188=COLOUR_RGB ( '',0.7921568627450980005, 0.8196078431372548767, 0.9333333333333333481 ) ;
#47205=EDGE_LOOP ( 'NONE', ( #61807, #22741, #22334, #10145, #38440, #14868, #1299 ) ) ;
#47218=VERTEX_POINT ( 'NONE', #6916 ) ;
#47259=DIRECTION ( 'NONE',  ( 1.110223024625156294E-16, 3.697785493223491743E-32, -1.000000000000000000 ) ) ;
#47353=ORIENTED_EDGE ( 'NONE', *, *, #28010, .T. ) ;
#47384=LINE ( 'NONE', #14697, #52934 ) ;
#47392=SURFACE_STYLE_USAGE ( .BOTH. , #36512 ) ;
#47437=PLANE ( 'NONE',  #54511 ) ;
#47456=AXIS2_PLACEMENT_3D ( 'NONE', #37535, #16435, #36511 ) ;
#47472=CARTESIAN_POINT ( 'NONE',  ( -452.6627218934862071, 370.0000000000064233, -141.4497041420121661 ) ) ;
#47478=FACE_OUTER_BOUND ( 'NONE', #3264, .T. ) ;
#47486=( NAMED_UNIT ( * ) PLANE_ANGLE_UNIT ( ) SI_UNIT ( $, .RADIAN. ) );
#47493=VECTOR ( 'NONE', #2503, 1000.000000000000000 ) ;
#47530=EDGE_CURVE ( 'NONE', #20487, #59656, #12752, .T. ) ;
#47559=AXIS2_PLACEMENT_3D ( 'NONE', #15595, #63787, #32116 ) ;
#47570=CYLINDRICAL_SURFACE ( 'NONE', #11753, 5.000000000000004441 ) ;
#47597=CIRCLE ( 'NONE', #67871, 5.000000000000004441 ) ;
#47614=ORIENTED_EDGE ( 'NONE', *, *, #50356, .F. ) ;
#47616=DIRECTION ( 'NONE',  ( 1.850169831522831466E-16, -1.000000000000000000, -1.110223024625156294E-16 ) ) ;
#47623=CARTESIAN_POINT ( 'NONE',  ( -417.6627218934913230, 399.9999999999997726, 113.5502958579881891 ) ) ;
#47633=EDGE_CURVE ( 'NONE', #4404, #24527, #10538, .T. ) ;
#47658=DIRECTION ( 'NONE',  ( 1.000000000000000000, 1.387778780781446169E-16, 0.000000000000000000 ) ) ;
#47659=DIRECTION ( 'NONE',  ( 0.000000000000000000, 0.000000000000000000, -1.000000000000000000 ) ) ;
#47694=DIRECTION ( 'NONE',  ( -0.7071067811865475727, 0.000000000000000000, -0.7071067811865474617 ) ) ;
#47698=AXIS2_PLACEMENT_3D ( 'NONE', #43496, #38227, #33321 ) ;
#47699=EDGE_CURVE ( 'NONE', #3371, #36808, #54746, .T. ) ;
#47721=ORIENTED_EDGE ( 'NONE', *, *, #6848, .F. ) ;
#47734=VERTEX_POINT ( 'NONE', #58548 ) ;
#47750=CARTESIAN_POINT ( 'NONE',  ( 442.3372781065085064, 390.0000000000001137, -141.4497041420117398 ) ) ;
#47765=AXIS2_PLACEMENT_3D ( 'NONE', #13561, #60352, #3011 ) ;
#47787=EDGE_CURVE ( 'NONE', #9014, #7875, #37441, .T. ) ;
#47818=FACE_OUTER_BOUND ( 'NONE', #36008, .T. ) ;
#47873=EDGE_CURVE ( 'NONE', #42825, #46238, #32339, .T. ) ;
#47901=CIRCLE ( 'NONE', #68165, 5.000000000000170530 ) ;
#47904=CARTESIAN_POINT ( 'NONE',  ( 417.3372781065085633, 394.9999999999999432, 83.55029585798834546 ) ) ;
#47931=ADVANCED_FACE ( 'NONE', ( #55365 ), #66637, .F. ) ;
#47939=ORIENTED_EDGE ( 'NONE', *, *, #56875, .F. ) ;
#47955=EDGE_CURVE ( 'NONE', #22681, #59605, #60410, .T. ) ;
#47963=CARTESIAN_POINT ( 'NONE',  ( -452.6627218934859798, 400.0000000000064801, -111.4497041420121661 ) ) ;
#47987=AXIS2_PLACEMENT_3D ( 'NONE', #27415, #48853, #1748 ) ;
#47994=EDGE_CURVE ( 'NONE', #17392, #18081, #23385, .T. ) ;
#48004=AXIS2_PLACEMENT_3D ( 'NONE', #25421, #35962, #9231 ) ;
#48040=LINE ( 'NONE', #63891, #46549 ) ;
#48065=CARTESIAN_POINT ( 'NONE',  ( 50.98853755884145755, 388.0000000000065370, -123.9497041420120382 ) ) ;
#48080=VERTEX_POINT ( 'NONE', #57796 ) ;
#48093=CARTESIAN_POINT ( 'NONE',  ( 447.3372781065083359, 400.0000000000044338, 83.55029585798381220 ) ) ;
#48098=DIRECTION ( 'NONE',  ( 9.729521452151193035E-15, -5.551115123116034723E-17, 1.000000000000000000 ) ) ;
#48130=AXIS2_PLACEMENT_3D ( 'NONE', #32979, #12574, #18198 ) ;
#48156=PLANE ( 'NONE',  #48703 ) ;
#48169=CARTESIAN_POINT ( 'NONE',  ( 447.3372781065085064, 365.0000000000043769, 113.5502958579838122 ) ) ;
#48174=EDGE_CURVE ( 'NONE', #1784, #45368, #63820, .T. ) ;
#48181=CARTESIAN_POINT ( 'NONE',  ( 442.3372781065086201, 0.000000000000000000, 103.5502958579881749 ) ) ;
#48203=CARTESIAN_POINT ( 'NONE',  ( 414.4083459183741525, 394.9999999999999432, 80.62136366985377833 ) ) ;
#48205=FACE_OUTER_BOUND ( 'NONE', #15140, .T. ) ;
#48213=LINE ( 'NONE', #6369, #30469 ) ;
#48216=PLANE ( 'NONE',  #6746 ) ;
#48232=AXIS2_PLACEMENT_3D ( 'NONE', #18801, #50806, #51843 ) ;
#48239=ADVANCED_FACE ( 'NONE', ( #27071 ), #10548, .F. ) ;
#48256=EDGE_CURVE ( 'NONE', #11896, #55210, #61566, .T. ) ;
#48257=VERTEX_POINT ( 'NONE', #32023 ) ;
#48289=EDGE_LOOP ( 'NONE', ( #46676, #37920, #23515, #52610 ) ) ;
#48301=ORIENTED_EDGE ( 'NONE', *, *, #47633, .F. ) ;
#48343=ORIENTED_EDGE ( 'NONE', *, *, #34114, .T. ) ;
#48346=ORIENTED_EDGE ( 'NONE', *, *, #27286, .T. ) ;
#48365=( GEOMETRIC_REPRESENTATION_CONTEXT ( 3 ) GLOBAL_UNCERTAINTY_ASSIGNED_CONTEXT ( ( #14197 ) ) GLOBAL_UNIT_ASSIGNED_CONTEXT ( ( #36592, #31645, #30623 ) ) REPRESENTATION_CONTEXT ( 'NONE', 'WORKASPACE' ) );
#48368=EDGE_LOOP ( 'NONE', ( #53203, #64773, #20295, #16268, #14812, #13028, #19438, #43547, #47353, #30835 ) ) ;
#48373=CARTESIAN_POINT ( 'NONE',  ( 429.8372781065087906, 388.0000000000066507, -133.9497041420121377 ) ) ;
#48396=ORIENTED_EDGE ( 'NONE', *, *, #5050, .F. ) ;
#48409=CARTESIAN_POINT ( 'NONE',  ( -439.4229916354183842, 394.9999999999998295, -128.9497041420121093 ) ) ;
#48439=VERTEX_POINT ( 'NONE', #2108 ) ;
#48468=DIRECTION ( 'NONE',  ( 0.000000000000000000, -6.405132834375902056E-16, 1.000000000000000000 ) ) ;
#48475=ORIENTED_EDGE ( 'NONE', *, *, #16884, .T. ) ;
#48486=CARTESIAN_POINT ( 'NONE',  ( 0.000000000000000000, 0.000000000000000000, 113.5502958579881749 ) ) ;
#48488=VECTOR ( 'NONE', #33712, 1000.000000000000000 ) ;
#48500=EDGE_CURVE ( 'NONE', #51645, #46238, #29870, .T. ) ;
#48509=CARTESIAN_POINT ( 'NONE',  ( 437.3372781065085633, 400.0000000000000568, -136.4497041420118251 ) ) ;
#48515=PLANE ( 'NONE',  #907 ) ;
#48538=CARTESIAN_POINT ( 'NONE',  ( -444.3832201885272184, 394.6953840236894280, 96.77545299096836118 ) ) ;
#48543=CARTESIAN_POINT ( 'NONE',  ( -442.6627218934912662, 394.9999999999998295, 91.05029585798840230 ) ) ;
#48551=PRESENTATION_STYLE_ASSIGNMENT (( #53498 ) ) ;
#48555=DIRECTION ( 'NONE',  ( 9.729521028634720986E-15, -5.551115123125782702E-17, 1.000000000000000000 ) ) ;
#48584=EDGE_LOOP ( 'NONE', ( #31629, #32562, #8356, #8986, #52400, #3414, #50965, #64259 ) ) ;
#48632=ORIENTED_EDGE ( 'NONE', *, *, #15575, .F. ) ;
#48649=EDGE_CURVE ( 'NONE', #66845, #17049, #64642, .T. ) ;
#48651=ADVANCED_FACE ( 'NONE', ( #15760 ), #36880, .T. ) ;
#48663=( BOUNDED_CURVE ( )  B_SPLINE_CURVE ( 3, ( #28506, #49950, #32735, #48884 ),
 .UNSPECIFIED., .F., .F. ) 
 B_SPLINE_CURVE_WITH_KNOTS ( ( 4, 4 ),
 ( 1.570796326794911879, 3.141592653589817985 ),
 .UNSPECIFIED. ) 
 CURVE ( )  GEOMETRIC_REPRESENTATION_ITEM ( )  RATIONAL_B_SPLINE_CURVE ( ( 1.000000000000000000, 0.8047378541243627170, 0.8047378541243627170, 1.000000000000000000 ) ) 
 REPRESENTATION_ITEM ( '' )  );
#48667=DIRECTION ( 'NONE',  ( 1.020422603260505347E-14, -1.000000000000000000, -5.551115123125782702E-17 ) ) ;
#48674=PLANE ( 'NONE',  #46524 ) ;
#48685=DIRECTION ( 'NONE',  ( 1.000000000000000000, 1.232595164407830672E-32, -5.551115123125781716E-16 ) ) ;
#48703=AXIS2_PLACEMENT_3D ( 'NONE', #47472, #26727, #69284 ) ;
#48705=EDGE_CURVE ( 'NONE', #27359, #24527, #15419, .T. ) ;
#48709=EDGE_CURVE ( 'NONE', #55220, #5511, #260, .T. ) ;
#48747=PLANE ( 'NONE',  #55409 ) ;
#48773=CYLINDRICAL_SURFACE ( 'NONE', #55647, 4.999999999999990230 ) ;
#48795=EDGE_LOOP ( 'NONE', ( #36715, #51401, #35649, #68217 ) ) ;
#48813=EDGE_LOOP ( 'NONE', ( #6563, #9136, #63794, #38128 ) ) ;
#48815=ORIENTED_EDGE ( 'NONE', *, *, #63368, .T. ) ;
#48826=CARTESIAN_POINT ( 'NONE',  ( 429.8372781065085633, 400.0000000000000568, -128.9497041420118251 ) ) ;
#48830=DIRECTION ( 'NONE',  ( -4.270088556250601699E-16, -0.000000000000000000, -1.000000000000000000 ) ) ;
#48852=ORIENTED_EDGE ( 'NONE', *, *, #45618, .F. ) ;
#48853=DIRECTION ( 'NONE',  ( -0.000000000000000000, -6.405132834375902056E-16, 1.000000000000000000 ) ) ;
#48858=ADVANCED_FACE ( 'NONE', ( #2025 ), #32975, .T. ) ;
#48868=DIRECTION ( 'NONE',  ( -1.387778780781445922E-16, 1.000000000000000000, 0.000000000000000000 ) ) ;
#48878=AXIS2_PLACEMENT_3D ( 'NONE', #49620, #8732, #12354 ) ;
#48884=CARTESIAN_POINT ( 'NONE',  ( -447.6627218934912094, 389.9999999999997726, 108.5502958579879476 ) ) ;
#48885=VECTOR ( 'NONE', #13415, 1000.000000000000000 ) ;
#48899=CARTESIAN_POINT ( 'NONE',  ( 424.8372781065087906, 395.0000000000042064, 91.05029585798442326 ) ) ;
#48917=ORIENTED_EDGE ( 'NONE', *, *, #42458, .T. ) ;
#48919=ORIENTED_EDGE ( 'NONE', *, *, #16159, .F. ) ;
#48933=AXIS2_PLACEMENT_3D ( 'NONE', #39254, #34682, #60698 ) ;
#48963=DIRECTION ( 'NONE',  ( -0.7071067811865545671, 2.831068712794148784E-15, -0.7071067811865405783 ) ) ;
#48996=PRODUCT_DEFINITION_FORMATION_WITH_SPECIFIED_SOURCE ( 'ANY', '', #8064, .NOT_KNOWN. ) ;
#49016=ORIENTED_EDGE ( 'NONE', *, *, #33835, .F. ) ;
#49024=CARTESIAN_POINT ( 'NONE',  ( -452.6627218934913230, 1.665334536937734811E-13, 83.55029585798817493 ) ) ;
#49030=CARTESIAN_POINT ( 'NONE',  ( -452.6627218934860366, 395.0000000000064801, -136.4497041420121661 ) ) ;
#49056=EDGE_LOOP ( 'NONE', ( #54805, #69492, #48396, #14787 ) ) ;
#49061=EDGE_CURVE ( 'NONE', #64521, #61561, #6052, .T. ) ;
#49091=CARTESIAN_POINT ( 'NONE',  ( 445.3372781065086201, 217.8591479523844612, 78.55029585798806124 ) ) ;
#49125=DIRECTION ( 'NONE',  ( -1.850169831522831466E-16, 1.000000000000000000, 1.110223024625156294E-16 ) ) ;
#49146=VERTEX_POINT ( 'NONE', #56003 ) ;
#49150=VECTOR ( 'NONE', #19784, 1000.000000000000000 ) ;
#49188=DIRECTION ( 'NONE',  ( 0.000000000000000000, 0.000000000000000000, -1.000000000000000000 ) ) ;
#49208=EDGE_CURVE ( 'NONE', #43624, #7362, #61951, .T. ) ;
#49227=PLANE ( 'NONE',  #41998 ) ;
#49242=AXIS2_PLACEMENT_3D ( 'NONE', #42611, #8887, #51791 ) ;
#49246=CARTESIAN_POINT ( 'NONE',  ( -444.2280788262714282, 394.7493581867591388, 97.47888161141302987 ) ) ;
#49273=DIRECTION ( 'NONE',  ( 3.081487911019579554E-32, 1.000000000000000000, 3.469446951953612956E-17 ) ) ;
#49312=EDGE_CURVE ( 'NONE', #33778, #22804, #65877, .T. ) ;
#49325=ORIENTED_EDGE ( 'NONE', *, *, #20546, .F. ) ;
#49353=CARTESIAN_POINT ( 'NONE',  ( -417.6627218934913230, 179.4906275429376308, 111.5502958579881749 ) ) ;
#49361=DIRECTION ( 'NONE',  ( -1.000000000000000000, -6.405132834375901070E-16, -5.170250902511168442E-32 ) ) ;
#49373=EDGE_CURVE ( 'NONE', #68802, #58622, #52100, .T. ) ;
#49385=PLANE ( 'NONE',  #37420 ) ;
#49396=PLANE ( 'NONE',  #43571 ) ;
#49400=ORIENTED_EDGE ( 'NONE', *, *, #30439, .F. ) ;
#49406=ORIENTED_EDGE ( 'NONE', *, *, #52357, .F. ) ;
#49426=VECTOR ( 'NONE', #56476, 1000.000000000000000 ) ;
#49435=EDGE_CURVE ( 'NONE', #61415, #47218, #67596, .T. ) ;
#49439=ORIENTED_EDGE ( 'NONE', *, *, #60611, .F. ) ;
#49453=CARTESIAN_POINT ( 'NONE',  ( -442.6627218934913799, 394.9999999999998295, -125.1412729879898791 ) ) ;
#49462=DIRECTION ( 'NONE',  ( -1.850169831522831466E-16, 1.000000000000000000, 1.110223024625156294E-16 ) ) ;
#49465=EDGE_LOOP ( 'NONE', ( #24479, #18, #13108, #54156 ) ) ;
#49477=ADVANCED_FACE ( 'NONE', ( #37993 ), #32377, .T. ) ;
#49486=FACE_OUTER_BOUND ( 'NONE', #9626, .T. ) ;
#49509=EDGE_CURVE ( 'NONE', #9149, #18081, #28992, .T. ) ;
#49544=DIRECTION ( 'NONE',  ( -1.000000000000000000, -1.334402673828311860E-15, -8.547026380416719758E-31 ) ) ;
#49571=ORIENTED_EDGE ( 'NONE', *, *, #49975, .F. ) ;
#49592=CARTESIAN_POINT ( 'NONE',  ( -442.6627218934918915, 395.0000000000064801, -136.4497041420121661 ) ) ;
#49604=ORIENTED_EDGE ( 'NONE', *, *, #60568, .T. ) ;
#49606=AXIS2_PLACEMENT_3D ( 'NONE', #12742, #23989, #23644 ) ;
#49620=CARTESIAN_POINT ( 'NONE',  ( -442.6627218934913230, 1.665334536937734811E-13, 103.5502958579881749 ) ) ;
#49625=EDGE_CURVE ( 'NONE', #41874, #36015, #15421, .T. ) ;
#49649=DIRECTION ( 'NONE',  ( 1.387778780781445922E-16, -1.000000000000000000, -1.232595164407830946E-32 ) ) ;
#49736=ORIENTED_EDGE ( 'NONE', *, *, #43957, .T. ) ;
#49752=DIRECTION ( 'NONE',  ( -1.387778780781446169E-16, 1.000000000000000000, 3.469446951953615421E-17 ) ) ;
#49769=AXIS2_PLACEMENT_3D ( 'NONE', #21536, #42982, #26485 ) ;
#49795=CARTESIAN_POINT ( 'NONE',  ( -447.6627218934913230, 399.9999999999997726, 103.5502958579881891 ) ) ;
#49815=CARTESIAN_POINT ( 'NONE',  ( -422.6627218934918915, 395.0000000000064801, -116.4497041420121377 ) ) ;
#49845=LINE ( 'NONE', #12578, #58856 ) ;
#49893=EDGE_LOOP ( 'NONE', ( #804, #4708, #37612, #20729 ) ) ;
#49927=EDGE_CURVE ( 'NONE', #41538, #67458, #36886, .T. ) ;
#49939=ORIENTED_EDGE ( 'NONE', *, *, #10089, .T. ) ;
#49950=CARTESIAN_POINT ( 'NONE',  ( -445.5916540816259044, 394.9999999999998863, 106.4792280461225715 ) ) ;
#49968=AXIS2_PLACEMENT_3D ( 'NONE', #38496, #63854, #32526 ) ;
#49975=EDGE_CURVE ( 'NONE', #24702, #19058, #23829, .T. ) ;
#49985=ORIENTED_EDGE ( 'NONE', *, *, #10558, .T. ) ;
#50001=LINE ( 'NONE', #11670, #13788 ) ;
#50007=FILL_AREA_STYLE_COLOUR ( '', #46492 ) ;
#50033=ORIENTED_EDGE ( 'NONE', *, *, #67580, .T. ) ;
#50044=DIRECTION ( 'NONE',  ( 1.387778780781446169E-16, -1.000000000000000000, -3.469446951953615421E-17 ) ) ;
#50059=ORIENTED_EDGE ( 'NONE', *, *, #26188, .T. ) ;
#50094=CARTESIAN_POINT ( 'NONE',  ( -447.6627218934914367, 389.9999999999954525, 108.5502958579925235 ) ) ;
#50097=DIRECTION ( 'NONE',  ( 1.337618101958020291E-16, 0.000000000000000000, -1.000000000000000000 ) ) ;
#50107=EDGE_CURVE ( 'NONE', #51413, #8171, #21765, .T. ) ;
#50110=ADVANCED_FACE ( 'NONE', ( #27261 ), #16371, .F. ) ;
#50133=VECTOR ( 'NONE', #11343, 1000.000000000000000 ) ;
#50182=ORIENTED_EDGE ( 'NONE', *, *, #66972, .F. ) ;
#50213=EDGE_CURVE ( 'NONE', #59106, #32147, #67160, .T. ) ;
#50317=AXIS2_PLACEMENT_3D ( 'NONE', #44823, #50097, #29679 ) ;
#50356=EDGE_CURVE ( 'NONE', #47218, #8003, #55940, .T. ) ;
#50374=VECTOR ( 'NONE', #61862, 1000.000000000000000 ) ;
#50383=MECHANICAL_DESIGN_GEOMETRIC_PRESENTATION_REPRESENTATION('',(#26819),#2130);
#50384=EDGE_LOOP ( 'NONE', ( #26763, #53555, #65758, #39779 ) ) ;
#50392=CARTESIAN_POINT ( 'NONE',  ( -447.6627218934912662, 369.9999999999998295, 113.5502958579880328 ) ) ;
#50399=CARTESIAN_POINT ( 'NONE',  ( 447.3372781065085633, 399.9999999999998863, 113.5502958579881891 ) ) ;
#50420=CARTESIAN_POINT ( 'NONE',  ( 112.3013380801408658, 400.0000000000066507, -123.9497041420121235 ) ) ;
#50469=ORIENTED_EDGE ( 'NONE', *, *, #33995, .T. ) ;
#50474=DIRECTION ( 'NONE',  ( -1.387778780781445922E-16, 1.000000000000000000, 1.232595164407830946E-32 ) ) ;
#50516=EDGE_LOOP ( 'NONE', ( #48346, #18229, #49604, #65427 ) ) ;
#50521=EDGE_CURVE ( 'NONE', #7387, #3371, #68616, .T. ) ;
#50530=CARTESIAN_POINT ( 'NONE',  ( 0.000000000000000000, 0.000000000000000000, 0.000000000000000000 ) ) ;
#50543=DIRECTION ( 'NONE',  ( 0.000000000000000000, 6.123233995736762338E-17, -1.000000000000000000 ) ) ;
#50557=VECTOR ( 'NONE', #52911, 1000.000000000000000 ) ;
#50568=ORIENTED_EDGE ( 'NONE', *, *, #27861, .F. ) ;
#50583=EDGE_CURVE ( 'NONE', #13335, #57503, #12243, .T. ) ;
#50586=PRESENTATION_STYLE_ASSIGNMENT (( #7338 ) ) ;
#50603=AXIS2_PLACEMENT_3D ( 'NONE', #63498, #6120, #53947 ) ;
#50607=LINE ( 'NONE', #2771, #62332 ) ;
#50636=ORIENTED_EDGE ( 'NONE', *, *, #64543, .F. ) ;
#50679=LINE ( 'NONE', #35198, #47493 ) ;
#50700=CARTESIAN_POINT ( 'NONE',  ( -417.6627218934913230, 179.4906275429376308, -146.4497041420118819 ) ) ;
#50752=CARTESIAN_POINT ( 'NONE',  ( 429.8372781065087338, 388.0000000000066507, -128.9497041420121093 ) ) ;
#50774=ORIENTED_EDGE ( 'NONE', *, *, #6435, .F. ) ;
#50792=CARTESIAN_POINT ( 'NONE',  ( -452.6627218934914367, 399.9999999999998863, -146.4497041420118251 ) ) ;
#50806=DIRECTION ( 'NONE',  ( -1.001915251000354105E-14, 1.000000000000000000, -5.551115123125782702E-17 ) ) ;
#50814=CARTESIAN_POINT ( 'NONE',  ( -422.6627218934913799, 394.9999999999998295, -116.4497041420117824 ) ) ;
#50815=ORIENTED_EDGE ( 'NONE', *, *, #68866, .T. ) ;
#50833=CARTESIAN_POINT ( 'NONE',  ( -417.6627218934913230, 219.4906275429376308, -146.4497041420118819 ) ) ;
#50853=DIRECTION ( 'NONE',  ( 1.000000000000000000, 2.465190328815660250E-32, 1.671219923253722421E-63 ) ) ;
#50885=EDGE_CURVE ( 'NONE', #15022, #22933, #35004, .T. ) ;
#50888=ORIENTED_EDGE ( 'NONE', *, *, #39553, .T. ) ;
#50891=EDGE_CURVE ( 'NONE', #52445, #42554, #23758, .T. ) ;
#50899=ORIENTED_EDGE ( 'NONE', *, *, #20631, .F. ) ;
#50931=VERTEX_POINT ( 'NONE', #37069 ) ;
#50937=CARTESIAN_POINT ( 'NONE',  ( 417.3372781065086201, 399.9999999999998863, 113.5502958579881891 ) ) ;
#50940=VECTOR ( 'NONE', #12247, 1000.000000000000000 ) ;
#50950=VERTEX_POINT ( 'NONE', #58510 ) ;
#50955=CARTESIAN_POINT ( 'NONE',  ( 442.3372781065089612, 390.0000000000074465, -141.4497041420121377 ) ) ;
#50958=ORIENTED_EDGE ( 'NONE', *, *, #15343, .T. ) ;
#50965=ORIENTED_EDGE ( 'NONE', *, *, #41772, .T. ) ;
#50974=CARTESIAN_POINT ( 'NONE',  ( -439.4229916354182706, 400.0000000000064801, 91.05029585798840230 ) ) ;
#50981=B_SPLINE_CURVE_WITH_KNOTS ( 'NONE', 3,
 ( #162, #11064, #52929, #869, #64537, #17027, #32527, #38145, #59585, #5448 ),
 .UNSPECIFIED., .F., .F.,
 ( 4, 2, 2, 2, 4 ),
 ( 0.004323147273503695660, 0.005401969756752221172, 0.006480792240000747551, 0.007559614723249273062, 0.008638437206497798573 ),
 .UNSPECIFIED. ) ;
#51050=DIRECTION ( 'NONE',  ( -0.7071067811865475727, 4.529112861587823989E-16, -0.7071067811865475727 ) ) ;
#51065=ORIENTED_EDGE ( 'NONE', *, *, #14295, .F. ) ;
#51073=CARTESIAN_POINT ( 'NONE',  ( -439.4229916354185548, 400.0000000000021032, 96.05029585799300662 ) ) ;
#51074=VERTEX_POINT ( 'NONE', #16304 ) ;
#51117=PLANE ( 'NONE',  #2601 ) ;
#51120=DIRECTION ( 'NONE',  ( 9.109522253334613014E-16, 1.000000000000000000, -3.889846672687432470E-31 ) ) ;
#51137=AXIS2_PLACEMENT_3D ( 'NONE', #6630, #54807, #17525 ) ;
#51138=FACE_OUTER_BOUND ( 'NONE', #34305, .T. ) ;
#51164=LINE ( 'NONE', #56786, #34767 ) ;
#51186=CARTESIAN_POINT ( 'NONE',  ( -447.6627218934913230, 399.9999999999997726, 83.55029585798818914 ) ) ;
#51214=ORIENTED_EDGE ( 'NONE', *, *, #46004, .F. ) ;
#51229=DIRECTION ( 'NONE',  ( -9.729521028634720986E-15, 5.551115123125782702E-17, -1.000000000000000000 ) ) ;
#51244=CARTESIAN_POINT ( 'NONE',  ( -442.6627218934912662, 394.9999999999998295, 92.24186470396634263 ) ) ;
#51257=VECTOR ( 'NONE', #7695, 1000.000000000000000 ) ;
#51261=DIRECTION ( 'NONE',  ( 2.921639538487254261E-16, 1.134144525784205431E-35, 1.000000000000000000 ) ) ;
#51267=EDGE_CURVE ( 'NONE', #13791, #36942, #30678, .T. ) ;
#51321=ORIENTED_EDGE ( 'NONE', *, *, #27286, .F. ) ;
#51350=ORIENTED_EDGE ( 'NONE', *, *, #33944, .T. ) ;
#51354=CARTESIAN_POINT ( 'NONE',  ( -450.6627218934913230, 217.8591479523843475, 78.55029585798814651 ) ) ;
#51357=CARTESIAN_POINT ( 'NONE',  ( 429.8372781065086770, 400.0000000000109708, 101.0502958579843948 ) ) ;
#51393=ADVANCED_FACE ( 'NONE', ( #48205 ), #379, .F. ) ;
#51401=ORIENTED_EDGE ( 'NONE', *, *, #39554, .T. ) ;
#51413=VERTEX_POINT ( 'NONE', #33457 ) ;
#51416=FILL_AREA_STYLE ('',( #50007 ) ) ;
#51457=DIRECTION ( 'NONE',  ( -1.000000000000000000, -1.001918046209079887E-14, 9.729495617646301779E-15 ) ) ;
#51468=ORIENTED_EDGE ( 'NONE', *, *, #44417, .F. ) ;
#51489=UNCERTAINTY_MEASURE_WITH_UNIT (LENGTH_MEASURE( 1.000000000000000082E-05 ), #8038, 'distance_accuracy_value', 'NONE');
#51490=ADVANCED_FACE ( 'NONE', ( #33096 ), #1084, .F. ) ;
#51491=FACE_OUTER_BOUND ( 'NONE', #26026, .T. ) ;
#51519=EDGE_LOOP ( 'NONE', ( #37452, #14399, #48917, #11341 ) ) ;
#51535=ORIENTED_EDGE ( 'NONE', *, *, #51917, .T. ) ;
#51538=AXIS2_PLACEMENT_3D ( 'NONE', #5915, #60083, #42533 ) ;
#51541=DIRECTION ( 'NONE',  ( -1.000000000000000000, -1.387778780781446908E-16, 0.000000000000000000 ) ) ;
#51568=EDGE_CURVE ( 'NONE', #1887, #56564, #26014, .T. ) ;
#51608=ORIENTED_EDGE ( 'NONE', *, *, #45343, .F. ) ;
#51642=EDGE_LOOP ( 'NONE', ( #41557, #30941, #5187, #33961 ) ) ;
#51644=FILL_AREA_STYLE_COLOUR ( '', #67808 ) ;
#51645=VERTEX_POINT ( 'NONE', #52722 ) ;
#51714=FACE_OUTER_BOUND ( 'NONE', #3854, .T. ) ;
#51742=CARTESIAN_POINT ( 'NONE',  ( -430.1627218934916073, 394.9999999999956231, 91.05029585799256608 ) ) ;
#51743=VECTOR ( 'NONE', #20303, 1000.000000000000000 ) ;
#51753=EDGE_LOOP ( 'NONE', ( #59560, #51350, #14440, #54590 ) ) ;
#51791=DIRECTION ( 'NONE',  ( -1.000000000000000000, 0.000000000000000000, 0.000000000000000000 ) ) ;
#51812=AXIS2_PLACEMENT_3D ( 'NONE', #50752, #24029, #55327 ) ;
#51842=ORIENTED_EDGE ( 'NONE', *, *, #49509, .T. ) ;
#51843=DIRECTION ( 'NONE',  ( -1.387778780781398344E-15, 0.000000000000000000, -1.000000000000000000 ) ) ;
#51862=VERTEX_POINT ( 'NONE', #35014 ) ;
#51865=EDGE_CURVE ( 'NONE', #17049, #14174, #55250, .T. ) ;
#51903=B_SPLINE_CURVE_WITH_KNOTS ( 'NONE', 3,
 ( #9936, #31389, #22558, #22910, #1107, #33123, #65128, #39104, #17272, #44002 ),
 .UNSPECIFIED., .F., .F.,
 ( 4, 2, 2, 2, 4 ),
 ( 0.000000000000000000, 0.001080786818375976174, 0.002161573636751952347, 0.003242360455127928521, 0.004323147273503904695 ),
 .UNSPECIFIED. ) ;
#51904=CARTESIAN_POINT ( 'NONE',  ( -435.1627218934913799, 399.9999999999998295, 96.05029585798821756 ) ) ;
#51914=CARTESIAN_POINT ( 'NONE',  ( -442.6627218934918915, 394.9999999999998295, -136.4497041420123367 ) ) ;
#51917=EDGE_CURVE ( 'NONE', #11940, #5635, #58868, .T. ) ;
#51940=CARTESIAN_POINT ( 'NONE',  ( -447.6627218934912662, 369.9999999999998295, 108.5502958579877060 ) ) ;
#51945=VERTEX_POINT ( 'NONE', #36745 ) ;
#51947=EDGE_LOOP ( 'NONE', ( #9659, #39456, #66339, #49325 ) ) ;
#51957=EDGE_CURVE ( 'NONE', #8171, #2857, #10011, .T. ) ;
#51973=FACE_OUTER_BOUND ( 'NONE', #66292, .T. ) ;
#52037=CARTESIAN_POINT ( 'NONE',  ( 447.3372781065086201, 400.0000000000044338, 113.5502958579838122 ) ) ;
#52045=AXIS2_PLACEMENT_3D ( 'NONE', #16448, #64986, #53024 ) ;
#52053=ORIENTED_EDGE ( 'NONE', *, *, #10223, .T. ) ;
#52070=DIRECTION ( 'NONE',  ( -1.000000000000000000, -1.387778780781438033E-16, 0.000000000000000000 ) ) ;
#52100=LINE ( 'NONE', #9889, #56998 ) ;
#52124=AXIS2_PLACEMENT_3D ( 'NONE', #19044, #49649, #22938 ) ;
#52129=ORIENTED_EDGE ( 'NONE', *, *, #15323, .T. ) ;
#52131=ORIENTED_EDGE ( 'NONE', *, *, #47955, .T. ) ;
#52153=CARTESIAN_POINT ( 'NONE',  ( -447.6627218934916073, 369.9999999999953957, 108.5502958579925377 ) ) ;
#52163=VERTEX_POINT ( 'NONE', #65831 ) ;
#52164=ADVANCED_FACE ( 'NONE', ( #54188 ), #17626, .F. ) ;
#52224=FACE_OUTER_BOUND ( 'NONE', #36047, .T. ) ;
#52232=DIRECTION ( 'NONE',  ( -4.270088556250601699E-16, -0.000000000000000000, -1.000000000000000000 ) ) ;
#52250=EDGE_CURVE ( 'NONE', #53656, #29332, #67230, .T. ) ;
#52255=ORIENTED_EDGE ( 'NONE', *, *, #46307, .T. ) ;
#52268=CARTESIAN_POINT ( 'NONE',  ( 429.8372781065087338, 395.0000000000042633, 96.05029585798436642 ) ) ;
#52269=LINE ( 'NONE', #19924, #62683 ) ;
#52285=VECTOR ( 'NONE', #18515, 1000.000000000000000 ) ;
#52290=DIRECTION ( 'NONE',  ( 0.7071067811865408004, -2.275957200481570908E-15, -0.7071067811865543451 ) ) ;
#52334=DIRECTION ( 'NONE',  ( -1.001915251000354105E-14, 1.000000000000000000, -5.551115123125782702E-17 ) ) ;
#52335=ADVANCED_FACE ( 'NONE', ( #68913 ), #26368, .F. ) ;
#52342=LINE ( 'NONE', #24243, #57579 ) ;
#52357=EDGE_CURVE ( 'NONE', #5511, #20487, #30270, .T. ) ;
#52372=ORIENTED_EDGE ( 'NONE', *, *, #67996, .F. ) ;
#52377=CARTESIAN_POINT ( 'NONE',  ( 447.3372781065083927, 395.0000000000043769, 83.55029585798381220 ) ) ;
#52391=DIRECTION ( 'NONE',  ( -7.703719777548943412E-34, 1.479221584281240009E-31, -1.000000000000000000 ) ) ;
#52400=ORIENTED_EDGE ( 'NONE', *, *, #51957, .T. ) ;
#52422=ORIENTED_EDGE ( 'NONE', *, *, #58661, .F. ) ;
#52445=VERTEX_POINT ( 'NONE', #33021 ) ;
#52499=CARTESIAN_POINT ( 'NONE',  ( 107.3013380801408658, 400.0000000000066507, -128.9497041420121093 ) ) ;
#52532=EDGE_LOOP ( 'NONE', ( #726, #5084, #60319, #58229, #3167, #14647, #28090 ) ) ;
#52561=VECTOR ( 'NONE', #61110, 1000.000000000000000 ) ;
#52582=DIRECTION ( 'NONE',  ( 0.000000000000000000, 6.123233995736762338E-17, -1.000000000000000000 ) ) ;
#52587=DIRECTION ( 'NONE',  ( -1.387778780781445429E-16, 1.000000000000000000, 3.081487911019577365E-33 ) ) ;
#52598=CARTESIAN_POINT ( 'NONE',  ( -445.5916540816261318, 394.9999999999995453, -139.3786363301466054 ) ) ;
#52610=ORIENTED_EDGE ( 'NONE', *, *, #19611, .F. ) ;
#52623=STYLED_ITEM ( 'NONE', ( #21088 ), #64062 ) ;
#52639=EDGE_CURVE ( 'NONE', #49146, #7569, #68827, .T. ) ;
#52640=LINE ( 'NONE', #63553, #1422 ) ;
#52647=ORIENTED_EDGE ( 'NONE', *, *, #12388, .F. ) ;
#52648=ADVANCED_FACE ( 'NONE', ( #51973 ), #56919, .F. ) ;
#52667=CARTESIAN_POINT ( 'NONE',  ( 442.3372781065085633, 370.0000000000001137, -146.4497041420116830 ) ) ;
#52704=ORIENTED_EDGE ( 'NONE', *, *, #18818, .F. ) ;
#52715=CARTESIAN_POINT ( 'NONE',  ( -450.6627218934913230, 217.8591479523843475, 78.55029585798814651 ) ) ;
#52717=DIRECTION ( 'NONE',  ( -1.000000000000000000, -1.001918046209079887E-14, 9.729495617646301779E-15 ) ) ;
#52722=CARTESIAN_POINT ( 'NONE',  ( -452.6627218934913230, 399.9999999999997726, 78.55029585798818914 ) ) ;
#52723=EDGE_CURVE ( 'NONE', #20392, #48439, #46693, .T. ) ;
#52738=PLANE ( 'NONE',  #26237 ) ;
#52781=EDGE_LOOP ( 'NONE', ( #59376, #37561, #6360, #13917, #47034, #9780, #21817 ) ) ;
#52791=AXIS2_PLACEMENT_3D ( 'NONE', #19537, #36410, #52582 ) ;
#52849=CARTESIAN_POINT ( 'NONE',  ( -417.6627218934916073, 397.0710678118612691, 78.55029585799223923 ) ) ;
#52851=ORIENTED_EDGE ( 'NONE', *, *, #13200, .T. ) ;
#52863=ORIENTED_EDGE ( 'NONE', *, *, #15489, .T. ) ;
#52874=VECTOR ( 'NONE', #65046, 1000.000000000000000 ) ;
#52911=DIRECTION ( 'NONE',  ( 1.000000000000000000, 1.387778780781445676E-16, -1.110223024625156294E-16 ) ) ;
#52929=CARTESIAN_POINT ( 'NONE',  ( -444.3832201885271616, 394.6953840236894280, -129.6748612749917129 ) ) ;
#52931=CYLINDRICAL_SURFACE ( 'NONE', #69139, 5.000000000000004441 ) ;
#52934=VECTOR ( 'NONE', #31237, 1000.000000000000000 ) ;
#52970=ORIENTED_EDGE ( 'NONE', *, *, #22943, .F. ) ;
#52973=EDGE_LOOP ( 'NONE', ( #20104, #53244, #6315, #12005 ) ) ;
#52984=ORIENTED_EDGE ( 'NONE', *, *, #50213, .F. ) ;
#53003=DIRECTION ( 'NONE',  ( -0.7071067811865405783, -7.105427357601001070E-15, 0.7071067811865545671 ) ) ;
#53024=DIRECTION ( 'NONE',  ( -1.000000000000000000, 0.000000000000000000, 0.000000000000000000 ) ) ;
#53077=CARTESIAN_POINT ( 'NONE',  ( 412.3372781065086201, 400.0000000000000568, -146.4497041420118251 ) ) ;
#53092=ORIENTED_EDGE ( 'NONE', *, *, #48705, .F. ) ;
#53101=EDGE_CURVE ( 'NONE', #20867, #5511, #52342, .T. ) ;
#53117=CARTESIAN_POINT ( 'NONE',  ( 429.8372781065084496, 400.0000000000042633, 96.05029585798401115 ) ) ;
#53124=EDGE_LOOP ( 'NONE', ( #13916, #9563, #61752, #57394 ) ) ;
#53130=ORIENTED_EDGE ( 'NONE', *, *, #43591, .F. ) ;
#53141=ORIENTED_EDGE ( 'NONE', *, *, #16250, .F. ) ;
#53163=MECHANICAL_DESIGN_GEOMETRIC_PRESENTATION_REPRESENTATION('',(#36372),#21736);
#53192=ADVANCED_FACE ( 'NONE', ( #21702 ), #43151, .T. ) ;
#53202=ADVANCED_FACE ( 'NONE', ( #20326 ), #36860, .T. ) ;
#53203=ORIENTED_EDGE ( 'NONE', *, *, #534, .F. ) ;
#53209=DIRECTION ( 'NONE',  ( -1.850169831522831466E-16, 1.000000000000000000, 1.110223024625156294E-16 ) ) ;
#53231=EDGE_LOOP ( 'NONE', ( #9271, #65433, #36859, #40386, #56315, #65991, #52129, #60706, #33013, #66826, #25559, #57919, #25001, #27373, #50774 ) ) ;
#53235=CARTESIAN_POINT ( 'NONE',  ( 412.3372781065085633, 179.4906275429376024, -144.4497041420117682 ) ) ;
#53244=ORIENTED_EDGE ( 'NONE', *, *, #44386, .F. ) ;
#53245=ORIENTED_EDGE ( 'NONE', *, *, #67684, .T. ) ;
#53258=CARTESIAN_POINT ( 'NONE',  ( -452.6627218934912662, 399.9999999999953957, 113.5502958579925661 ) ) ;
#53272=DIRECTION ( 'NONE',  ( 9.899279560275165216E-15, -1.665334536937735057E-16, 1.000000000000000000 ) ) ;
#53352=EDGE_LOOP ( 'NONE', ( #49985, #67121, #35476, #63123 ) ) ;
#53362=VECTOR ( 'NONE', #61317, 1000.000000000000000 ) ;
#53382=LINE ( 'NONE', #10482, #6999 ) ;
#53399=EDGE_CURVE ( 'NONE', #11896, #4675, #7279, .T. ) ;
#53407=AXIS2_PLACEMENT_3D ( 'NONE', #66617, #51120, #7866 ) ;
#53429=EDGE_CURVE ( 'NONE', #60705, #57073, #55098, .T. ) ;
#53446=ORIENTED_EDGE ( 'NONE', *, *, #46473, .T. ) ;
#53460=CARTESIAN_POINT ( 'NONE',  ( 440.2662102946430309, 394.9999999999997726, 106.4792280461226994 ) ) ;
#53461=LINE ( 'NONE', #48181, #5823 ) ;
#53477=EDGE_LOOP ( 'NONE', ( #13302, #54828, #38502, #3929 ) ) ;
#53498=SURFACE_STYLE_USAGE ( .BOTH. , #65466 ) ;
#53499=CARTESIAN_POINT ( 'NONE',  ( -417.6627218934913230, 219.4906275429376308, 111.5502958579881749 ) ) ;
#53539=CARTESIAN_POINT ( 'NONE',  ( 447.3372781065085633, 177.8591479523844612, -111.4497041420119388 ) ) ;
#53550=DIRECTION ( 'NONE',  ( 1.387778780781445429E-16, -1.000000000000000000, -3.081487911019577365E-33 ) ) ;
#53553=FACE_OUTER_BOUND ( 'NONE', #30532, .T. ) ;
#53555=ORIENTED_EDGE ( 'NONE', *, *, #51568, .F. ) ;
#53559=LINE ( 'NONE', #16965, #59097 ) ;
#53561=EDGE_LOOP ( 'NONE', ( #49571, #3400, #7449, #25665 ) ) ;
#53573=VECTOR ( 'NONE', #9666, 1000.000000000000000 ) ;
#53577=CARTESIAN_POINT ( 'NONE',  ( 112.3013380801406811, 400.0000000000077307, 101.0502958579874644 ) ) ;
#53578=ORIENTED_EDGE ( 'NONE', *, *, #69235, .T. ) ;
#53586=CARTESIAN_POINT ( 'NONE',  ( -447.6627218934913230, 394.9999999999998295, 108.5502958579881181 ) ) ;
#53635=EDGE_LOOP ( 'NONE', ( #62632, #69437, #30288, #19768 ) ) ;
#53656=VERTEX_POINT ( 'NONE', #27588 ) ;
#53719=COLOUR_RGB ( '',0.7921568627450980005, 0.8196078431372548767, 0.9333333333333333481 ) ;
#53750=CARTESIAN_POINT ( 'NONE',  ( 412.3372781065086770, 0.000000000000000000, 113.5502958579881749 ) ) ;
#53763=CARTESIAN_POINT ( 'NONE',  ( 412.3372781065085633, 400.0000000000000568, -146.4497041420118535 ) ) ;
#53788=AXIS2_PLACEMENT_3D ( 'NONE', #25596, #25246, #47031 ) ;
#53845=CARTESIAN_POINT ( 'NONE',  ( 112.3013380801408658, 388.0000000000065938, -128.9497041420121093 ) ) ;
#53846=DIRECTION ( 'NONE',  ( -7.703719777548945123E-34, -1.479221584281240009E-31, 1.000000000000000000 ) ) ;
#53872=EDGE_LOOP ( 'NONE', ( #56676, #9372, #45378 ) ) ;
#53882=EDGE_CURVE ( 'NONE', #55296, #22681, #27504, .T. ) ;
#53889=CARTESIAN_POINT ( 'NONE',  ( 412.3372781065085633, 400.0000000000000568, -146.4497041420118535 ) ) ;
#53899=LINE ( 'NONE', #21906, #50133 ) ;
#53901=EDGE_CURVE ( 'NONE', #41002, #42064, #44024, .T. ) ;
#53935=DIRECTION ( 'NONE',  ( 1.000000000000000000, 0.000000000000000000, -2.921639538487254261E-16 ) ) ;
#53947=DIRECTION ( 'NONE',  ( 0.7071067811865475727, 0.000000000000000000, 0.7071067811865474617 ) ) ;
#53966=CARTESIAN_POINT ( 'NONE',  ( 417.3372781065086201, 399.9999999999998863, 108.5502958579882034 ) ) ;
#54003=DIRECTION ( 'NONE',  ( 1.110515250991959028E-16, 1.000000000000000000, 1.110223024625156294E-16 ) ) ;
#54050=EDGE_CURVE ( 'NONE', #50931, #2896, #20337, .T. ) ;
#54055=ORIENTED_EDGE ( 'NONE', *, *, #56725, .F. ) ;
#54097=CARTESIAN_POINT ( 'NONE',  ( 429.8372781065087338, 394.9999999999999432, 91.05029585798857283 ) ) ;
#54111=LINE ( 'NONE', #5596, #52874 ) ;
#54123=ADVANCED_FACE ( 'NONE', ( #25973 ), #36872, .T. ) ;
#54132=ORIENTED_EDGE ( 'NONE', *, *, #43837, .T. ) ;
#54156=ORIENTED_EDGE ( 'NONE', *, *, #35889, .T. ) ;
#54182=SURFACE_STYLE_FILL_AREA ( #33469 ) ;
#54188=FACE_OUTER_BOUND ( 'NONE', #31616, .T. ) ;
#54211=CARTESIAN_POINT ( 'NONE',  ( 442.3372781065085064, 390.0000000000001137, -141.4497041420117398 ) ) ;
#54225=DIRECTION ( 'NONE',  ( -9.109522253334613014E-16, -1.000000000000000000, 3.889846672687432470E-31 ) ) ;
#54227=AXIS2_PLACEMENT_3D ( 'NONE', #64621, #41791, #63592 ) ;
#54252=CARTESIAN_POINT ( 'NONE',  ( -435.1627218934913799, 399.9999999999998295, 96.05029585798821756 ) ) ;
#54254=AXIS2_PLACEMENT_3D ( 'NONE', #38495, #11758, #27239 ) ;
#54261=ORIENTED_EDGE ( 'NONE', *, *, #20391, .T. ) ;
#54267=PLANE ( 'NONE',  #61483 ) ;
#54269=VECTOR ( 'NONE', #25696, 1000.000000000000000 ) ;
#54279=VECTOR ( 'NONE', #35676, 1000.000000000000000 ) ;
#54297=EDGE_CURVE ( 'NONE', #62102, #44967, #5979, .T. ) ;
#54328=ORIENTED_EDGE ( 'NONE', *, *, #50213, .T. ) ;
#54334=CARTESIAN_POINT ( 'NONE',  ( -417.6627218934913230, 397.0710678118655323, 78.55029585798810388 ) ) ;
#54349=ORIENTED_EDGE ( 'NONE', *, *, #50521, .F. ) ;
#54386=EDGE_CURVE ( 'NONE', #17804, #16476, #58751, .T. ) ;
#54392=CARTESIAN_POINT ( 'NONE',  ( 412.3372781065086201, 399.9999999999998863, 113.5502958579881891 ) ) ;
#54407=ORIENTED_EDGE ( 'NONE', *, *, #53882, .T. ) ;
#54414=VERTEX_POINT ( 'NONE', #3393 ) ;
#54429=VECTOR ( 'NONE', #12495, 1000.000000000000000 ) ;
#54464=FILL_AREA_STYLE_COLOUR ( '', #47188 ) ;
#54473=ORIENTED_EDGE ( 'NONE', *, *, #29645, .F. ) ;
#54476=VERTEX_POINT ( 'NONE', #16356 ) ;
#54511=AXIS2_PLACEMENT_3D ( 'NONE', #38193, #20723, #65638 ) ;
#54557=DIRECTION ( 'NONE',  ( 1.020422603260505347E-14, -1.000000000000000000, -5.551115123125782702E-17 ) ) ;
#54568=ORIENTED_EDGE ( 'NONE', *, *, #2053, .F. ) ;
#54575=CARTESIAN_POINT ( 'NONE',  ( -439.4229916354185548, 395.0000000000065370, -133.9497041420121377 ) ) ;
#54590=ORIENTED_EDGE ( 'NONE', *, *, #16803, .T. ) ;
#54591=CARTESIAN_POINT ( 'NONE',  ( -439.4229916354182706, 388.0000000000064801, -123.9497041420119530 ) ) ;
#54632=CARTESIAN_POINT ( 'NONE',  ( 412.3372781065085633, 179.4906275429376024, -144.4497041420117682 ) ) ;
#54643=ORIENTED_EDGE ( 'NONE', *, *, #56724, .F. ) ;
#54655=ORIENTED_EDGE ( 'NONE', *, *, #16969, .F. ) ;
#54679=LINE ( 'NONE', #6507, #35573 ) ;
#54709=DIRECTION ( 'NONE',  ( -1.000000000000000000, 1.232595164407830946E-32, 7.703719777548943412E-34 ) ) ;
#54732=VECTOR ( 'NONE', #16561, 1000.000000000000000 ) ;
#54746=LINE ( 'NONE', #23104, #24475 ) ;
#54754=DIRECTION ( 'NONE',  ( -3.344045254895050726E-17, -1.000000000000000000, 0.000000000000000000 ) ) ;
#54805=ORIENTED_EDGE ( 'NONE', *, *, #26324, .T. ) ;
#54807=DIRECTION ( 'NONE',  ( -0.7071067811865474617, 9.422489238170280455E-15, 0.7071067811865475727 ) ) ;
#54808=FILL_AREA_STYLE ('',( #58694 ) ) ;
#54828=ORIENTED_EDGE ( 'NONE', *, *, #69547, .F. ) ;
#54903=ORIENTED_EDGE ( 'NONE', *, *, #15008, .F. ) ;
#54939=VERTEX_POINT ( 'NONE', #795 ) ;
#54966=LINE ( 'NONE', #64836, #36535 ) ;
#55087=( NAMED_UNIT ( * ) SI_UNIT ( $, .STERADIAN. ) SOLID_ANGLE_UNIT ( ) );
#55098=LINE ( 'NONE', #43498, #2595 ) ;
#55111=CARTESIAN_POINT ( 'NONE',  ( 112.3013380801406385, 400.0000000000077307, 96.05029585798746439 ) ) ;
#55132=VERTEX_POINT ( 'NONE', #43609 ) ;
#55141=ORIENTED_EDGE ( 'NONE', *, *, #8130, .F. ) ;
#55155=ADVANCED_FACE ( 'NONE', ( #1062 ), #49227, .F. ) ;
#55173=CARTESIAN_POINT ( 'NONE',  ( -417.6627218934915504, 399.9999999999957367, 78.55029585799222502 ) ) ;
#55191=ADVANCED_FACE ( 'NONE', ( #16877 ), #59438, .F. ) ;
#55194=VERTEX_POINT ( 'NONE', #33774 ) ;
#55199=AXIS2_PLACEMENT_3D ( 'NONE', #58931, #16379, #26251 ) ;
#55209=ORIENTED_EDGE ( 'NONE', *, *, #27891, .T. ) ;
#55210=VERTEX_POINT ( 'NONE', #17223 ) ;
#55212=DIRECTION ( 'NONE',  ( 1.110223024625156294E-16, 3.697785493223491743E-32, -1.000000000000000000 ) ) ;
#55215=DIRECTION ( 'NONE',  ( 0.000000000000000000, 1.232595164407830672E-32, -1.000000000000000000 ) ) ;
#55220=VERTEX_POINT ( 'NONE', #6683 ) ;
#55237=ORIENTED_EDGE ( 'NONE', *, *, #23355, .T. ) ;
#55250=CIRCLE ( 'NONE', #207, 5.000000000000004441 ) ;
#55251=CARTESIAN_POINT ( 'NONE',  ( 312.3372781065084496, 394.9999999999999432, -21.44970414201177888 ) ) ;
#55269=LINE ( 'NONE', #17996, #21756 ) ;
#55296=VERTEX_POINT ( 'NONE', #28846 ) ;
#55303=ORIENTED_EDGE ( 'NONE', *, *, #45213, .T. ) ;
#55327=DIRECTION ( 'NONE',  ( -1.000000000000000000, 0.000000000000000000, 0.000000000000000000 ) ) ;
#55355=DIRECTION ( 'NONE',  ( 1.000000000000000000, 1.850550996349095901E-16, 1.228197773518735191E-20 ) ) ;
#55358=EDGE_CURVE ( 'NONE', #38637, #17049, #66491, .T. ) ;
#55365=FACE_OUTER_BOUND ( 'NONE', #50384, .T. ) ;
#55409=AXIS2_PLACEMENT_3D ( 'NONE', #585, #22036, #7618 ) ;
#55439=CARTESIAN_POINT ( 'NONE',  ( 445.3372781065085633, 177.8591479523844612, -111.4497041420119388 ) ) ;
#55452=LINE ( 'NONE', #7635, #18499 ) ;
#55468=ORIENTED_EDGE ( 'NONE', *, *, #27009, .T. ) ;
#55478=CARTESIAN_POINT ( 'NONE',  ( -442.6627218934913230, 399.9999999999997726, 108.5502958579881891 ) ) ;
#55488=COLOUR_RGB ( '',0.7921568627450980005, 0.8196078431372548767, 0.9333333333333333481 ) ;
#55491=LINE ( 'NONE', #13626, #62270 ) ;
#55502=CARTESIAN_POINT ( 'NONE',  ( -447.6627218934913799, 369.9999999999998295, -141.4497041420117966 ) ) ;
#55511=FILL_AREA_STYLE ('',( #44959 ) ) ;
#55524=DIRECTION ( 'NONE',  ( 1.000000000000000000, 1.387778780781445922E-16, 0.000000000000000000 ) ) ;
#55574=CARTESIAN_POINT ( 'NONE',  ( 442.3372781065085633, 367.0710678118653050, 108.5502958579886439 ) ) ;
#55575=EDGE_LOOP ( 'NONE', ( #10836, #24737, #20781, #7513 ) ) ;
#55579=VERTEX_POINT ( 'NONE', #20184 ) ;
#55602=CARTESIAN_POINT ( 'NONE',  ( -422.6627218934914367, 0.000000000000000000, -141.4497041420118535 ) ) ;
#55622=LINE ( 'NONE', #34878, #59003 ) ;
#55647=AXIS2_PLACEMENT_3D ( 'NONE', #48093, #21715, #22068 ) ;
#55656=VECTOR ( 'NONE', #14592, 1000.000000000000000 ) ;
#55676=MECHANICAL_DESIGN_GEOMETRIC_PRESENTATION_REPRESENTATION('',(#13521),#42508);
#55680=ORIENTED_EDGE ( 'NONE', *, *, #14306, .F. ) ;
#55722=DIRECTION ( 'NONE',  ( 0.000000000000000000, 6.123233995736870806E-17, -1.000000000000000000 ) ) ;
#55753=LINE ( 'NONE', #2296, #56968 ) ;
#55778=DIRECTION ( 'NONE',  ( -6.405132834375898112E-16, 1.000000000000000000, 1.281026566875181792E-15 ) ) ;
#55795=PRODUCT_DEFINITION_SHAPE ( 'NONE', 'NONE',  #46499 ) ;
#55815=FACE_OUTER_BOUND ( 'NONE', #53231, .T. ) ;
#55827=DIRECTION ( 'NONE',  ( -0.7071067811865476838, -1.110223024625156294E-16, -0.7071067811865474617 ) ) ;
#55881=ORIENTED_EDGE ( 'NONE', *, *, #37008, .F. ) ;
#55884=DIRECTION ( 'NONE',  ( 1.387778780781445922E-16, -1.000000000000000000, -1.232595164407830946E-32 ) ) ;
#55896=CARTESIAN_POINT ( 'NONE',  ( -452.6627218934862071, 370.0000000000064233, -141.4497041420121661 ) ) ;
#55906=ORIENTED_EDGE ( 'NONE', *, *, #23118, .T. ) ;
#55940=CIRCLE ( 'NONE', #60406, 5.000000000000004441 ) ;
#55944=AXIS2_PLACEMENT_3D ( 'NONE', #60648, #45861, #67332 ) ;
#55983=FACE_OUTER_BOUND ( 'NONE', #35797, .T. ) ;
#55987=CARTESIAN_POINT ( 'NONE',  ( -435.1627218934888788, 400.0000000000064801, -128.9497041420092387 ) ) ;
#55999=EDGE_CURVE ( 'NONE', #41255, #17804, #56702, .T. ) ;
#56003=CARTESIAN_POINT ( 'NONE',  ( -447.6627218934916073, 369.9999999999953957, 108.5502958579925377 ) ) ;
#56010=EDGE_LOOP ( 'NONE', ( #50182, #4877, #11973, #48301 ) ) ;
#56022=PLANE ( 'NONE',  #1158 ) ;
#56059=VERTEX_POINT ( 'NONE', #11565 ) ;
#56099=DIRECTION ( 'NONE',  ( 1.000000000000000000, 1.387778780781445676E-16, -1.110223024625156294E-16 ) ) ;
#56105=ORIENTED_EDGE ( 'NONE', *, *, #32851, .T. ) ;
#56206=CARTESIAN_POINT ( 'NONE',  ( 429.8372781065086201, 388.0000000000109708, 96.05029585798438063 ) ) ;
#56221=( NAMED_UNIT ( * ) SI_UNIT ( $, .STERADIAN. ) SOLID_ANGLE_UNIT ( ) );
#56241=CARTESIAN_POINT ( 'NONE',  ( -452.6627218934913799, 0.000000000000000000, -111.4497041420118251 ) ) ;
#56243=EDGE_CURVE ( 'NONE', #36104, #20970, #68138, .T. ) ;
#56279=FACE_OUTER_BOUND ( 'NONE', #4953, .T. ) ;
#56292=DIRECTION ( 'NONE',  ( -1.000000000000000000, -1.850550996349095901E-16, -1.228197773518735191E-20 ) ) ;
#56299=EDGE_CURVE ( 'NONE', #22995, #42825, #24539, .T. ) ;
#56315=ORIENTED_EDGE ( 'NONE', *, *, #59864, .F. ) ;
#56387=ORIENTED_EDGE ( 'NONE', *, *, #2306, .T. ) ;
#56401=DIRECTION ( 'NONE',  ( -1.850169831522831466E-16, 1.000000000000000000, 1.110223024625156294E-16 ) ) ;
#56448=DIRECTION ( 'NONE',  ( -1.000000000000000000, -1.001918829714556097E-14, 9.899279560275163638E-15 ) ) ;
#56458=CARTESIAN_POINT ( 'NONE',  ( -442.6627218934913230, 394.9999999999998295, -123.9497041420119530 ) ) ;
#56476=DIRECTION ( 'NONE',  ( 6.405132834375898112E-16, -1.000000000000000000, 1.396592535537253184E-14 ) ) ;
#56549=ORIENTED_EDGE ( 'NONE', *, *, #51267, .F. ) ;
#56551=MECHANICAL_DESIGN_GEOMETRIC_PRESENTATION_REPRESENTATION('',(#25141),#27357);
#56564=VERTEX_POINT ( 'NONE', #20613 ) ;
#56676=ORIENTED_EDGE ( 'NONE', *, *, #20982, .T. ) ;
#56702=LINE ( 'NONE', #60809, #17389 ) ;
#56714=CIRCLE ( 'NONE', #5031, 5.000000000000060396 ) ;
#56724=EDGE_CURVE ( 'NONE', #29739, #51945, #20885, .T. ) ;
#56725=EDGE_CURVE ( 'NONE', #13975, #910, #24192, .T. ) ;
#56774=EDGE_CURVE ( 'NONE', #55132, #13975, #15951, .T. ) ;
#56782=DIRECTION ( 'NONE',  ( -1.000000000000000000, -1.001918046209079887E-14, 9.729495617646301779E-15 ) ) ;
#56786=CARTESIAN_POINT ( 'NONE',  ( -444.4229916354184979, 388.0000000000064233, 96.05029585798874336 ) ) ;
#56788=CARTESIAN_POINT ( 'NONE',  ( -447.6627218934913230, 367.0710678118653050, 108.5502958579877202 ) ) ;
#56792=CARTESIAN_POINT ( 'NONE',  ( 447.3372781065085633, 399.9999999999998863, 83.55029585798818914 ) ) ;
#56811=FACE_OUTER_BOUND ( 'NONE', #2713, .T. ) ;
#56816=AXIS2_PLACEMENT_3D ( 'NONE', #33674, #66391, #18875 ) ;
#56822=EDGE_CURVE ( 'NONE', #135, #51413, #60599, .T. ) ;
#56825=CARTESIAN_POINT ( 'NONE',  ( 445.3372781065085633, 217.8591479523844612, -111.4497041420119388 ) ) ;
#56854=CARTESIAN_POINT ( 'NONE',  ( 447.3372781065086201, 370.0000000000043769, 108.5502958579838264 ) ) ;
#56863=AXIS2_PLACEMENT_3D ( 'NONE', #46015, #29839, #26298 ) ;
#56875=EDGE_CURVE ( 'NONE', #46890, #48257, #54966, .T. ) ;
#56878=ORIENTED_EDGE ( 'NONE', *, *, #2306, .F. ) ;
#56919=PLANE ( 'NONE',  #22718 ) ;
#56926=PRESENTATION_STYLE_ASSIGNMENT (( #23528 ) ) ;
#56927=ORIENTED_EDGE ( 'NONE', *, *, #6427, .T. ) ;
#56968=VECTOR ( 'NONE', #56099, 1000.000000000000000 ) ;
#56970=AXIS2_PLACEMENT_3D ( 'NONE', #40232, #55355, #2260 ) ;
#56998=VECTOR ( 'NONE', #8856, 1000.000000000000000 ) ;
#57006=FACE_OUTER_BOUND ( 'NONE', #55575, .T. ) ;
#57007=ORIENTED_EDGE ( 'NONE', *, *, #28276, .T. ) ;
#57049=ORIENTED_EDGE ( 'NONE', *, *, #21990, .F. ) ;
#57073=VERTEX_POINT ( 'NONE', #51354 ) ;
#57078=CARTESIAN_POINT ( 'NONE',  ( -430.1627218934915504, 399.9999999999998863, -123.9497041420119530 ) ) ;
#57155=CARTESIAN_POINT ( 'NONE',  ( 112.3013380801408232, 388.0000000000077307, 101.0502958579874644 ) ) ;
#57169=ADVANCED_FACE ( 'NONE', ( #32313 ), #58677, .F. ) ;
#57222=CARTESIAN_POINT ( 'NONE',  ( 447.3372781065085633, 217.8591479523844612, -111.4497041420119388 ) ) ;
#57228=DIRECTION ( 'NONE',  ( 0.000000000000000000, 6.123233995736761105E-17, -1.000000000000000000 ) ) ;
#57237=CARTESIAN_POINT ( 'NONE',  ( -447.6627218934913230, 399.9999999999997726, 83.55029585798818914 ) ) ;
#57266=FILL_AREA_STYLE ('',( #14358 ) ) ;
#57332=ORIENTED_EDGE ( 'NONE', *, *, #66400, .F. ) ;
#57352=EDGE_CURVE ( 'NONE', #57676, #62102, #12164, .T. ) ;
#57394=ORIENTED_EDGE ( 'NONE', *, *, #43655, .T. ) ;
#57418=CARTESIAN_POINT ( 'NONE',  ( 107.3013380801407237, 395.0000000000010232, 96.05029585798752123 ) ) ;
#57451=DIRECTION ( 'NONE',  ( -0.000000000000000000, -6.405132834375902056E-16, 1.000000000000000000 ) ) ;
#57474=VERTEX_POINT ( 'NONE', #35705 ) ;
#57481=ORIENTED_EDGE ( 'NONE', *, *, #4654, .T. ) ;
#57490=ADVANCED_FACE ( 'NONE', ( #56811 ), #8630, .F. ) ;
#57503=VERTEX_POINT ( 'NONE', #67713 ) ;
#57509=DIRECTION ( 'NONE',  ( 0.000000000000000000, 1.000000000000000000, 0.000000000000000000 ) ) ;
#57519=CARTESIAN_POINT ( 'NONE',  ( -444.4229916354184979, 394.6798985497181889, -128.9497041420121093 ) ) ;
#57578=ORIENTED_EDGE ( 'NONE', *, *, #36205, .F. ) ;
#57579=VECTOR ( 'NONE', #19995, 1000.000000000000000 ) ;
#57580=EDGE_CURVE ( 'NONE', #22806, #35973, #46583, .T. ) ;
#57601=EDGE_CURVE ( 'NONE', #66548, #55194, #46940, .T. ) ;
#57617=DIRECTION ( 'NONE',  ( 1.000000000000000000, 0.000000000000000000, -0.000000000000000000 ) ) ;
#57628=SURFACE_STYLE_FILL_AREA ( #14707 ) ;
#57640=CARTESIAN_POINT ( 'NONE',  ( 440.2662102946430878, 395.0000000000000568, -139.3786363301463211 ) ) ;
#57642=DIRECTION ( 'NONE',  ( -3.081487911019579554E-32, -1.000000000000000000, -3.469446951953612956E-17 ) ) ;
#57669=DIRECTION ( 'NONE',  ( 0.7071067811865408004, -2.275957200481570908E-15, -0.7071067811865543451 ) ) ;
#57676=VERTEX_POINT ( 'NONE', #26519 ) ;
#57677=DIRECTION ( 'NONE',  ( 0.000000000000000000, -6.123233995736870806E-17, 1.000000000000000000 ) ) ;
#57705=LINE ( 'NONE', #68598, #6037 ) ;
#57712=( GEOMETRIC_REPRESENTATION_CONTEXT ( 3 ) GLOBAL_UNCERTAINTY_ASSIGNED_CONTEXT ( ( #17744 ) ) GLOBAL_UNIT_ASSIGNED_CONTEXT ( ( #46815, #47486, #46462 ) ) REPRESENTATION_CONTEXT ( 'NONE', 'WORKASPACE' ) );
#57725=EDGE_CURVE ( 'NONE', #56059, #54414, #15620, .T. ) ;
#57735=ORIENTED_EDGE ( 'NONE', *, *, #49208, .F. ) ;
#57736=PLANE ( 'NONE',  #47146 ) ;
#57755=DIRECTION ( 'NONE',  ( -1.850371928290090422E-16, 1.000000000000000000, 1.110223024625156171E-16 ) ) ;
#57788=ORIENTED_EDGE ( 'NONE', *, *, #24838, .T. ) ;
#57796=CARTESIAN_POINT ( 'NONE',  ( -417.6627218934913230, 219.4906275429376308, 113.5502958579881749 ) ) ;
#57810=ADVANCED_FACE ( 'NONE', ( #37756 ), #6087, .F. ) ;
#57847=LINE ( 'NONE', #42357, #53573 ) ;
#57866=CARTESIAN_POINT ( 'NONE',  ( 414.4083459183738114, 395.0000000000040927, 80.62136366984962876 ) ) ;
#57873=DIRECTION ( 'NONE',  ( 1.000000000000000000, 1.387778780781445429E-16, 0.000000000000000000 ) ) ;
#57896=ORIENTED_EDGE ( 'NONE', *, *, #5050, .T. ) ;
#57916=FACE_OUTER_BOUND ( 'NONE', #24806, .T. ) ;
#57919=ORIENTED_EDGE ( 'NONE', *, *, #65039, .T. ) ;
#57922=LINE ( 'NONE', #31200, #12257 ) ;
#57944=DIRECTION ( 'NONE',  ( -7.703719777548945123E-34, -1.479221584281240009E-31, 1.000000000000000000 ) ) ;
#57953=LINE ( 'NONE', #69190, #41135 ) ;
#57996=ADVANCED_FACE ( 'NONE', ( #61985 ), #45466, .T. ) ;
#57998=ORIENTED_EDGE ( 'NONE', *, *, #16773, .F. ) ;
#58015=VECTOR ( 'NONE', #26115, 1000.000000000000000 ) ;
#58051=CARTESIAN_POINT ( 'NONE',  ( 442.3372781065089612, 367.0710678118721262, -141.4497041420121377 ) ) ;
#58065=CARTESIAN_POINT ( 'NONE',  ( -439.4229916354183274, 394.9999999999998295, 96.05029585798874336 ) ) ;
#58085=ORIENTED_EDGE ( 'NONE', *, *, #12162, .F. ) ;
#58092=CIRCLE ( 'NONE', #20989, 5.000000000000004441 ) ;
#58100=VECTOR ( 'NONE', #13706, 1000.000000000000000 ) ;
#58124=DIRECTION ( 'NONE',  ( 1.000000000000000000, 0.000000000000000000, -1.697894969632809662E-16 ) ) ;
#58185=VERTEX_POINT ( 'NONE', #4971 ) ;
#58206=DIRECTION ( 'NONE',  ( 1.000000000000000000, 1.387778780781444936E-16, 0.000000000000000000 ) ) ;
#58208=ORIENTED_EDGE ( 'NONE', *, *, #10223, .F. ) ;
#58217=LINE ( 'NONE', #31830, #1538 ) ;
#58229=ORIENTED_EDGE ( 'NONE', *, *, #48174, .T. ) ;
#58240=ORIENTED_EDGE ( 'NONE', *, *, #42935, .T. ) ;
#58243=ORIENTED_EDGE ( 'NONE', *, *, #22795, .T. ) ;
#58262=DIRECTION ( 'NONE',  ( -7.703719777548945123E-34, -1.479221584281240009E-31, 1.000000000000000000 ) ) ;
#58263=ORIENTED_EDGE ( 'NONE', *, *, #14752, .T. ) ;
#58284=ORIENTED_EDGE ( 'NONE', *, *, #48709, .T. ) ;
#58314=ORIENTED_EDGE ( 'NONE', *, *, #50521, .T. ) ;
#58344=EDGE_CURVE ( 'NONE', #6017, #36914, #43283, .T. ) ;
#58350=LINE ( 'NONE', #68242, #64739 ) ;
#58363=ORIENTED_EDGE ( 'NONE', *, *, #54297, .F. ) ;
#58398=ORIENTED_EDGE ( 'NONE', *, *, #65109, .F. ) ;
#58425=CARTESIAN_POINT ( 'NONE',  ( 412.3372781065086201, 399.9999999999998863, 78.55029585798826020 ) ) ;
#58450=SURFACE_SIDE_STYLE ('',( #68668 ) ) ;
#58462=EDGE_LOOP ( 'NONE', ( #13295, #69001, #29821, #39822 ) ) ;
#58468=LINE ( 'NONE', #42973, #62238 ) ;
#58508=EDGE_CURVE ( 'NONE', #36015, #5564, #58350, .T. ) ;
#58510=CARTESIAN_POINT ( 'NONE',  ( 447.3372781065085064, 364.9999999999990905, 113.5502958579887007 ) ) ;
#58513=DIRECTION ( 'NONE',  ( -6.939198835768237954E-16, -1.000000000000000000, -6.106226635438359986E-16 ) ) ;
#58516=VECTOR ( 'NONE', #60175, 999.9999999999998863 ) ;
#58548=CARTESIAN_POINT ( 'NONE',  ( -442.6627218934912662, 394.9999999999998295, 103.5502958579880612 ) ) ;
#58597=AXIS2_PLACEMENT_3D ( 'NONE', #39213, #12475, #30383 ) ;
#58612=CLOSED_SHELL ( 'NONE', ( #65266, #58823, #28280, #29320, #12014, #9011 ) ) ;
#58622=VERTEX_POINT ( 'NONE', #61050 ) ;
#58661=EDGE_CURVE ( 'NONE', #5564, #32464, #60702, .T. ) ;
#58672=ORIENTED_EDGE ( 'NONE', *, *, #25257, .T. ) ;
#58677=PLANE ( 'NONE',  #7312 ) ;
#58694=FILL_AREA_STYLE_COLOUR ( '', #53719 ) ;
#58738=DIRECTION ( 'NONE',  ( -6.405132834375897126E-16, 1.000000000000000000, 0.000000000000000000 ) ) ;
#58750=ORIENTED_EDGE ( 'NONE', *, *, #49927, .T. ) ;
#58751=CIRCLE ( 'NONE', #63295, 5.000000000000004441 ) ;
#58823=ADVANCED_FACE ( 'NONE', ( #52224 ), #14593, .T. ) ;
#58836=CARTESIAN_POINT ( 'NONE',  ( 445.3372781065086201, 217.8591479523844612, 78.55029585798806124 ) ) ;
#58856=VECTOR ( 'NONE', #65704, 1000.000000000000000 ) ;
#58866=FACE_OUTER_BOUND ( 'NONE', #27847, .T. ) ;
#58868=LINE ( 'NONE', #31804, #35036 ) ;
#58874=EDGE_LOOP ( 'NONE', ( #64741, #69285, #39182, #35816 ) ) ;
#58931=CARTESIAN_POINT ( 'NONE',  ( -447.6627218934914367, 399.9999999999998863, -136.4497041420118251 ) ) ;
#58970=ADVANCED_FACE ( 'NONE', ( #39178 ), #60621, .F. ) ;
#59003=VECTOR ( 'NONE', #18336, 1000.000000000000000 ) ;
#59021=EDGE_LOOP ( 'NONE', ( #37788, #979, #38665, #13956 ) ) ;
#59043=( LENGTH_UNIT ( ) NAMED_UNIT ( * ) SI_UNIT ( .MILLI., .METRE. ) );
#59046=FACE_OUTER_BOUND ( 'NONE', #7378, .T. ) ;
#59051=EDGE_LOOP ( 'NONE', ( #33547, #14356, #41221, #68916 ) ) ;
#59068=EDGE_LOOP ( 'NONE', ( #45528, #57332, #9994, #40935 ) ) ;
#59072=PRESENTATION_STYLE_ASSIGNMENT (( #21442 ) ) ;
#59088=ORIENTED_EDGE ( 'NONE', *, *, #13298, .F. ) ;
#59090=CARTESIAN_POINT ( 'NONE',  ( 442.3372781065083927, 392.9289321881345813, 108.5502958579881465 ) ) ;
#59097=VECTOR ( 'NONE', #33170, 1000.000000000000000 ) ;
#59106=VERTEX_POINT ( 'NONE', #41931 ) ;
#59139=AXIS2_PLACEMENT_3D ( 'NONE', #45419, #51050, #66900 ) ;
#59169=ORIENTED_EDGE ( 'NONE', *, *, #27484, .F. ) ;
#59194=VECTOR ( 'NONE', #24059, 1000.000000000000000 ) ;
#59198=VECTOR ( 'NONE', #21929, 1000.000000000000000 ) ;
#59231=VERTEX_POINT ( 'NONE', #12582 ) ;
#59250=PLANE ( 'NONE',  #46609 ) ;
#59281=AXIS2_PLACEMENT_3D ( 'NONE', #48509, #21453, #42226 ) ;
#59306=ORIENTED_EDGE ( 'NONE', *, *, #44830, .T. ) ;
#59307=EDGE_LOOP ( 'NONE', ( #30316, #28217, #52647, #24562 ) ) ;
#59333=FACE_OUTER_BOUND ( 'NONE', #53352, .T. ) ;
#59376=ORIENTED_EDGE ( 'NONE', *, *, #32851, .F. ) ;
#59385=EDGE_CURVE ( 'NONE', #4870, #67714, #2342, .T. ) ;
#59386=VERTEX_POINT ( 'NONE', #61423 ) ;
#59403=LINE ( 'NONE', #11920, #37755 ) ;
#59431=DIRECTION ( 'NONE',  ( 1.000000000000000000, 0.000000000000000000, 0.000000000000000000 ) ) ;
#59438=CYLINDRICAL_SURFACE ( 'NONE', #43136, 5.000000000000060396 ) ;
#59484=PLANE ( 'NONE',  #44132 ) ;
#59521=CARTESIAN_POINT ( 'NONE',  ( 447.3372781065086201, 177.8591479523844612, 78.55029585798806124 ) ) ;
#59534=VECTOR ( 'NONE', #47259, 1000.000000000000000 ) ;
#59549=ORIENTED_EDGE ( 'NONE', *, *, #56774, .F. ) ;
#59552=DIRECTION ( 'NONE',  ( -3.344045254895050726E-17, -1.000000000000000000, -4.069049096960790458E-32 ) ) ;
#59560=ORIENTED_EDGE ( 'NONE', *, *, #42773, .T. ) ;
#59573=LINE ( 'NONE', #27930, #40598 ) ;
#59576=DIRECTION ( 'NONE',  ( -3.081487911019579554E-32, -1.000000000000000000, -3.469446951953612956E-17 ) ) ;
#59585=CARTESIAN_POINT ( 'NONE',  ( -442.9409111889697783, 394.9999999999998863, -132.5214871221317878 ) ) ;
#59605=VERTEX_POINT ( 'NONE', #34188 ) ;
#59627=ORIENTED_EDGE ( 'NONE', *, *, #23735, .T. ) ;
#59656=VERTEX_POINT ( 'NONE', #45773 ) ;
#59678=EDGE_CURVE ( 'NONE', #58185, #16629, #60554, .T. ) ;
#59713=CLOSED_SHELL ( 'NONE', ( #17044, #42169, #19483, #9832, #1687, #17972, #36985, #41724, #24077 ) ) ;
#59715=EDGE_CURVE ( 'NONE', #13434, #50950, #55622, .T. ) ;
#59728=PLANE ( 'NONE',  #51538 ) ;
#59737=ORIENTED_EDGE ( 'NONE', *, *, #7337, .F. ) ;
#59741=DIRECTION ( 'NONE',  ( 1.604841615724182956E-15, 1.000000000000000000, 1.604841615724182561E-15 ) ) ;
#59763=ORIENTED_EDGE ( 'NONE', *, *, #64543, .T. ) ;
#59781=CARTESIAN_POINT ( 'NONE',  ( -447.6627218934912094, 389.9999999999997726, 108.5502958579879476 ) ) ;
#59803=CARTESIAN_POINT ( 'NONE',  ( -444.1138056043201345, 394.7873829578389291, 97.81866361316865266 ) ) ;
#59819=CARTESIAN_POINT ( 'NONE',  ( 437.3372781065085633, 399.9999999999998863, 108.5502958579881891 ) ) ;
#59861=AXIS2_PLACEMENT_3D ( 'NONE', #43331, #54225, #32451 ) ;
#59864=EDGE_CURVE ( 'NONE', #20962, #57676, #23201, .T. ) ;
#59880=ORIENTED_EDGE ( 'NONE', *, *, #2948, .T. ) ;
#59899=PLANE ( 'NONE',  #33425 ) ;
#59914=FACE_OUTER_BOUND ( 'NONE', #19709, .T. ) ;
#59941=FACE_OUTER_BOUND ( 'NONE', #48368, .T. ) ;
#59971=DIRECTION ( 'NONE',  ( -3.417256381633830033E-15, -1.000000000000000000, -5.551115123125782702E-17 ) ) ;
#59974=( BOUNDED_CURVE ( )  B_SPLINE_CURVE ( 3, ( #10876, #32346, #678, #27048 ),
 .UNSPECIFIED., .F., .T. ) 
 B_SPLINE_CURVE_WITH_KNOTS ( ( 4, 4 ),
 ( -8.881784197001252323E-16, 1.570796326794896336 ),
 .UNSPECIFIED. ) 
 CURVE ( )  GEOMETRIC_REPRESENTATION_ITEM ( )  RATIONAL_B_SPLINE_CURVE ( ( 1.000000000000000000, 0.8047378541243649375, 0.8047378541243649375, 1.000000000000000000 ) ) 
 REPRESENTATION_ITEM ( '' )  );
#59997=CARTESIAN_POINT ( 'NONE',  ( 107.3013380801408658, 388.0000000000065938, -128.9497041420121093 ) ) ;
#60055=ORIENTED_EDGE ( 'NONE', *, *, #60568, .F. ) ;
#60058=VECTOR ( 'NONE', #57228, 1000.000000000000000 ) ;
#60063=DIRECTION ( 'NONE',  ( 1.000000000000000000, 0.000000000000000000, 0.000000000000000000 ) ) ;
#60065=EDGE_LOOP ( 'NONE', ( #12955, #23655, #45445, #34688 ) ) ;
#60083=DIRECTION ( 'NONE',  ( 1.232595164407830946E-32, 1.000000000000000000, -1.479221584281239571E-31 ) ) ;
#60087=ADVANCED_FACE ( 'NONE', ( #6579 ), #12208, .F. ) ;
#60167=DIRECTION ( 'NONE',  ( -4.270088556250601699E-16, -0.000000000000000000, -1.000000000000000000 ) ) ;
#60169=CARTESIAN_POINT ( 'NONE',  ( -440.1146514826276643, 395.0000000000064801, -133.9016337311479958 ) ) ;
#60175=DIRECTION ( 'NONE',  ( -0.7071067811865473507, 6.441404958702665783E-16, 0.7071067811865477948 ) ) ;
#60253=ADVANCED_FACE ( 'NONE', ( #42395 ), #52931, .T. ) ;
#60265=ORIENTED_EDGE ( 'NONE', *, *, #68894, .T. ) ;
#60319=ORIENTED_EDGE ( 'NONE', *, *, #44657, .T. ) ;
#60352=DIRECTION ( 'NONE',  ( -1.850371928290090422E-16, 1.000000000000000000, 1.110223024625156294E-16 ) ) ;
#60406=AXIS2_PLACEMENT_3D ( 'NONE', #29033, #50474, #2295 ) ;
#60410=CIRCLE ( 'NONE', #55944, 5.000000000000004441 ) ;
#60433=DIRECTION ( 'NONE',  ( 3.835731315158922607E-15, 1.000000000000000000, 5.551115123125782702E-17 ) ) ;
#60461=LINE ( 'NONE', #28810, #19007 ) ;
#60468=CARTESIAN_POINT ( 'NONE',  ( -447.6627218934889925, 395.0000000000064801, -141.4497041420092387 ) ) ;
#60477=SURFACE_SIDE_STYLE ('',( #14239 ) ) ;
#60480=CYLINDRICAL_SURFACE ( 'NONE', #47987, 5.000000000000004441 ) ;
#60506=CIRCLE ( 'NONE', #36912, 5.000000000000004441 ) ;
#60514=DIRECTION ( 'NONE',  ( -1.000000000000000000, -2.465190328815660250E-32, -1.671219923253722421E-63 ) ) ;
#60515=LINE ( 'NONE', #28867, #32350 ) ;
#60535=FACE_OUTER_BOUND ( 'NONE', #45719, .T. ) ;
#60543=VERTEX_POINT ( 'NONE', #61692 ) ;
#60554=LINE ( 'NONE', #1827, #48885 ) ;
#60562=CIRCLE ( 'NONE', #65027, 5.000000000000170530 ) ;
#60568=EDGE_CURVE ( 'NONE', #28396, #54939, #63079, .T. ) ;
#60590=CARTESIAN_POINT ( 'NONE',  ( -417.6627218934913230, 1.665334536937734811E-13, 113.5502958579881749 ) ) ;
#60599=LINE ( 'NONE', #54252, #16282 ) ;
#60611=EDGE_CURVE ( 'NONE', #59231, #16988, #24473, .T. ) ;
#60621=CYLINDRICAL_SURFACE ( 'NONE', #63486, 5.000000000000170530 ) ;
#60643=UNCERTAINTY_MEASURE_WITH_UNIT (LENGTH_MEASURE( 1.000000000000000082E-05 ), #59043, 'distance_accuracy_value', 'NONE');
#60648=CARTESIAN_POINT ( 'NONE',  ( -452.6627218934913799, 0.000000000000000000, -116.4497041420118393 ) ) ;
#60677=CARTESIAN_POINT ( 'NONE',  ( -439.4229916354183274, 400.0000000000064801, 96.05029585798874336 ) ) ;
#60698=DIRECTION ( 'NONE',  ( -1.000000000000000000, 0.000000000000000000, 0.000000000000000000 ) ) ;
#60702=LINE ( 'NONE', #28703, #2834 ) ;
#60705=VERTEX_POINT ( 'NONE', #17668 ) ;
#60706=ORIENTED_EDGE ( 'NONE', *, *, #9454, .T. ) ;
#60710=PLANE ( 'NONE',  #31800 ) ;
#60794=ORIENTED_EDGE ( 'NONE', *, *, #46887, .F. ) ;
#60799=FACE_OUTER_BOUND ( 'NONE', #67939, .T. ) ;
#60800=LINE ( 'NONE', #28450, #8670 ) ;
#60803=ADVANCED_FACE ( 'NONE', ( #14391 ), #41465, .F. ) ;
#60809=CARTESIAN_POINT ( 'NONE',  ( 112.3013380801408658, 388.0000000000065938, -133.9497041420121377 ) ) ;
#60817=( BOUNDED_CURVE ( )  B_SPLINE_CURVE ( 3, ( #25472, #30739, #62043, #36012 ),
 .UNSPECIFIED., .F., .F. ) 
 B_SPLINE_CURVE_WITH_KNOTS ( ( 4, 4 ),
 ( 3.140184917367546389E-16, 1.570796326794907882 ),
 .UNSPECIFIED. ) 
 CURVE ( )  GEOMETRIC_REPRESENTATION_ITEM ( )  RATIONAL_B_SPLINE_CURVE ( ( 1.000000000000000000, 0.8047378541243622729, 0.8047378541243622729, 1.000000000000000000 ) ) 
 REPRESENTATION_ITEM ( '' )  );
#60824=ORIENTED_EDGE ( 'NONE', *, *, #9847, .F. ) ;
#60833=DIRECTION ( 'NONE',  ( -1.000000000000000000, -2.922263668027335568E-20, -3.557538378468060822E-20 ) ) ;
#60867=AXIS2_PLACEMENT_3D ( 'NONE', #5023, #37042, #67685 ) ;
#60897=ORIENTED_EDGE ( 'NONE', *, *, #18364, .T. ) ;
#60971=ORIENTED_EDGE ( 'NONE', *, *, #27211, .F. ) ;
#60980=VERTEX_POINT ( 'NONE', #23122 ) ;
#60986=DIRECTION ( 'NONE',  ( 0.000000000000000000, 0.000000000000000000, 1.000000000000000000 ) ) ;
#61033=VECTOR ( 'NONE', #33480, 1000.000000000000000 ) ;
#61050=CARTESIAN_POINT ( 'NONE',  ( 412.3372781065086770, 0.000000000000000000, -146.4497041420118251 ) ) ;
#61094=ORIENTED_EDGE ( 'NONE', *, *, #29125, .F. ) ;
#61096=VECTOR ( 'NONE', #30804, 1000.000000000000000 ) ;
#61110=DIRECTION ( 'NONE',  ( 0.000000000000000000, -1.000000000000000000, -2.184185950696548891E-33 ) ) ;
#61144=( NAMED_UNIT ( * ) SI_UNIT ( $, .STERADIAN. ) SOLID_ANGLE_UNIT ( ) );
#61160=SURFACE_SIDE_STYLE ('',( #61508 ) ) ;
#61184=AXIS2_PLACEMENT_3D ( 'NONE', #5103, #43415, #47658 ) ;
#61187=VECTOR ( 'NONE', #6215, 1000.000000000000000 ) ;
#61232=CARTESIAN_POINT ( 'NONE',  ( -447.6627218934913799, 389.9999999999998295, -141.4497041420118535 ) ) ;
#61236=DIRECTION ( 'NONE',  ( -0.7071067811865474617, -9.058225723175622340E-16, 0.7071067811865474617 ) ) ;
#61278=VECTOR ( 'NONE', #31506, 1000.000000000000114 ) ;
#61291=ORIENTED_EDGE ( 'NONE', *, *, #10134, .T. ) ;
#61317=DIRECTION ( 'NONE',  ( -1.000000000000000000, 1.232595164407830946E-32, 7.703719777548943412E-34 ) ) ;
#61371=DIRECTION ( 'NONE',  ( 1.000000000000000000, 0.000000000000000000, 0.000000000000000000 ) ) ;
#61377=LINE ( 'NONE', #7222, #9168 ) ;
#61391=EDGE_CURVE ( 'NONE', #12220, #21613, #54679, .T. ) ;
#61415=VERTEX_POINT ( 'NONE', #19838 ) ;
#61423=CARTESIAN_POINT ( 'NONE',  ( -452.6627218934913799, 364.9999999999998295, -146.4497041420117966 ) ) ;
#61425=VECTOR ( 'NONE', #40066, 1000.000000000000000 ) ;
#61435=CARTESIAN_POINT ( 'NONE',  ( -450.6627218934913230, 177.8591479523843475, -111.4497041420117966 ) ) ;
#61483=AXIS2_PLACEMENT_3D ( 'NONE', #54632, #59552, #43720 ) ;
#61498=CARTESIAN_POINT ( 'NONE',  ( 50.98853755884145755, 400.0000000000065938, -123.9497041420120382 ) ) ;
#61508=SURFACE_STYLE_FILL_AREA ( #43914 ) ;
#61514=LINE ( 'NONE', #60468, #27468 ) ;
#61551=LINE ( 'NONE', #34831, #58100 ) ;
#61553=ADVANCED_FACE ( 'NONE', ( #10995 ), #64120, .T. ) ;
#61557=DIRECTION ( 'NONE',  ( 1.000000000000000000, -3.344045254895050726E-17, -0.000000000000000000 ) ) ;
#61561=VERTEX_POINT ( 'NONE', #15251 ) ;
#61566=CIRCLE ( 'NONE', #36866, 5.000000000000004441 ) ;
#61591=ORIENTED_EDGE ( 'NONE', *, *, #33835, .T. ) ;
#61598=DIRECTION ( 'NONE',  ( 1.000000000000000000, 2.117582368135750246E-20, -1.697742017499683849E-16 ) ) ;
#61636=ORIENTED_EDGE ( 'NONE', *, *, #62334, .T. ) ;
#61639=CARTESIAN_POINT ( 'NONE',  ( 417.3372781065091317, 395.0000000000065938, -116.4497041420121661 ) ) ;
#61642=EDGE_LOOP ( 'NONE', ( #61291, #58314, #19456, #63814 ) ) ;
#61680=CARTESIAN_POINT ( 'NONE',  ( 112.3013380801408658, 388.0000000000065938, -128.9497041420121093 ) ) ;
#61692=CARTESIAN_POINT ( 'NONE',  ( -442.6627218934913799, 394.9999999999998295, -132.7581352960343679 ) ) ;
#61694=EDGE_CURVE ( 'NONE', #15354, #42101, #33160, .T. ) ;
#61706=ORIENTED_EDGE ( 'NONE', *, *, #42586, .T. ) ;
#61717=FACE_OUTER_BOUND ( 'NONE', #22674, .T. ) ;
#61727=EDGE_LOOP ( 'NONE', ( #44799, #60265, #9093, #20010, #52704, #30175, #32807 ) ) ;
#61733=LINE ( 'NONE', #56458, #7398 ) ;
#61752=ORIENTED_EDGE ( 'NONE', *, *, #53429, .T. ) ;
#61759=CARTESIAN_POINT ( 'NONE',  ( 433.3728120124415568, 388.0000000000066507, -132.4852380479447902 ) ) ;
#61789=EDGE_CURVE ( 'NONE', #36104, #25372, #47901, .T. ) ;
#61807=ORIENTED_EDGE ( 'NONE', *, *, #10134, .F. ) ;
#61809=VECTOR ( 'NONE', #50044, 1000.000000000000000 ) ;
#61833=CARTESIAN_POINT ( 'NONE',  ( -442.6627218934914367, 399.9999999999998863, -141.4497041420118251 ) ) ;
#61848=ORIENTED_EDGE ( 'NONE', *, *, #44800, .F. ) ;
#61862=DIRECTION ( 'NONE',  ( -3.081487911019579554E-32, -1.000000000000000000, -3.469446951953612956E-17 ) ) ;
#61886=ORIENTED_EDGE ( 'NONE', *, *, #38417, .T. ) ;
#61933=VECTOR ( 'NONE', #57755, 1000.000000000000000 ) ;
#61937=DIRECTION ( 'NONE',  ( -1.000000000000000000, -1.001918046209079887E-14, 9.729495617646301779E-15 ) ) ;
#61951=LINE ( 'NONE', #24346, #69332 ) ;
#61962=ORIENTED_EDGE ( 'NONE', *, *, #6798, .F. ) ;
#61981=CARTESIAN_POINT ( 'NONE',  ( -442.9415673952017301, 394.9999999999997726, -125.3784793789377261 ) ) ;
#61985=FACE_OUTER_BOUND ( 'NONE', #53872, .T. ) ;
#62002=FACE_OUTER_BOUND ( 'NONE', #53124, .T. ) ;
#62020=LINE ( 'NONE', #35301, #59194 ) ;
#62043=CARTESIAN_POINT ( 'NONE',  ( -419.7337897053573670, 395.0000000000063665, -113.5207719538776558 ) ) ;
#62063=ORIENTED_EDGE ( 'NONE', *, *, #33995, .F. ) ;
#62080=EDGE_CURVE ( 'NONE', #12369, #19058, #55753, .T. ) ;
#62081=CARTESIAN_POINT ( 'NONE',  ( 437.3372781065086201, 0.000000000000000000, -136.4497041420118251 ) ) ;
#62102=VERTEX_POINT ( 'NONE', #20523 ) ;
#62141=CARTESIAN_POINT ( 'NONE',  ( 437.3372781065085633, 400.0000000000000568, -141.4497041420118251 ) ) ;
#62186=CIRCLE ( 'NONE', #47559, 5.000000000000004441 ) ;
#62195=DIRECTION ( 'NONE',  ( -1.000000000000000000, -1.387778780781446908E-16, 0.000000000000000000 ) ) ;
#62197=CYLINDRICAL_SURFACE ( 'NONE', #3460, 5.000000000000004441 ) ;
#62200=ORIENTED_EDGE ( 'NONE', *, *, #5234, .T. ) ;
#62227=VECTOR ( 'NONE', #3549, 1000.000000000000000 ) ;
#62238=VECTOR ( 'NONE', #21527, 1000.000000000000000 ) ;
#62248=CARTESIAN_POINT ( 'NONE',  ( 437.3372781065091885, 395.0000000000066507, -136.4497041420121661 ) ) ;
#62270=VECTOR ( 'NONE', #24200, 1000.000000000000000 ) ;
#62271=DIRECTION ( 'NONE',  ( -1.020422603260505347E-14, 1.000000000000000000, 5.551115123125782702E-17 ) ) ;
#62296=CARTESIAN_POINT ( 'NONE',  ( -447.6627218934913230, 1.665334536937734811E-13, 103.5502958579881749 ) ) ;
#62303=DIRECTION ( 'NONE',  ( 1.000000000000000000, 0.000000000000000000, -5.551115123125593376E-15 ) ) ;
#62305=ORIENTED_EDGE ( 'NONE', *, *, #1652, .T. ) ;
#62307=DIRECTION ( 'NONE',  ( 0.000000000000000000, 4.930380657631322689E-32, 1.000000000000000000 ) ) ;
#62318=VERTEX_POINT ( 'NONE', #45369 ) ;
#62332=VECTOR ( 'NONE', #40397, 1000.000000000000000 ) ;
#62334=EDGE_CURVE ( 'NONE', #46955, #20867, #61551, .T. ) ;
#62347=EDGE_LOOP ( 'NONE', ( #48919, #32996, #27712, #44845 ) ) ;
#62355=LINE ( 'NONE', #37332, #44460 ) ;
#62404=DIRECTION ( 'NONE',  ( -1.850371928290090422E-16, 1.000000000000000000, 1.110223024625156171E-16 ) ) ;
#62434=ORIENTED_EDGE ( 'NONE', *, *, #10466, .T. ) ;
#62453=DIRECTION ( 'NONE',  ( 0.7071067811865477948, -9.875400524329059797E-15, 0.7071067811865473507 ) ) ;
#62473=FACE_OUTER_BOUND ( 'NONE', #53477, .T. ) ;
#62482=DIRECTION ( 'NONE',  ( -3.330669073875466466E-14, 0.000000000000000000, -1.000000000000000000 ) ) ;
#62504=ADVANCED_FACE ( 'NONE', ( #41405 ), #36463, .F. ) ;
#62511=ORIENTED_EDGE ( 'NONE', *, *, #2568, .T. ) ;
#62530=VECTOR ( 'NONE', #29759, 1000.000000000000000 ) ;
#62535=DIRECTION ( 'NONE',  ( 1.000000000000000000, 1.387778780781445922E-16, 0.000000000000000000 ) ) ;
#62552=DIRECTION ( 'NONE',  ( 1.387778780781445429E-16, -1.000000000000000000, -3.081487911019577365E-33 ) ) ;
#62599=VECTOR ( 'NONE', #47616, 1000.000000000000000 ) ;
#62632=ORIENTED_EDGE ( 'NONE', *, *, #17130, .F. ) ;
#62642=LINE ( 'NONE', #63327, #46507 ) ;
#62663=VERTEX_POINT ( 'NONE', #5816 ) ;
#62676=( BOUNDED_CURVE ( )  B_SPLINE_CURVE ( 3, ( #44145, #66346, #23760, #38898 ),
 .UNSPECIFIED., .F., .F. ) 
 B_SPLINE_CURVE_WITH_KNOTS ( ( 4, 4 ),
 ( 1.570796326794884568, 3.141592653589783346 ),
 .UNSPECIFIED. ) 
 CURVE ( )  GEOMETRIC_REPRESENTATION_ITEM ( )  RATIONAL_B_SPLINE_CURVE ( ( 1.000000000000000000, 0.8047378541243644934, 0.8047378541243644934, 1.000000000000000000 ) ) 
 REPRESENTATION_ITEM ( '' )  );
#62677=VECTOR ( 'NONE', #57451, 1000.000000000000000 ) ;
#62683=VECTOR ( 'NONE', #41380, 1000.000000000000000 ) ;
#62712=DIRECTION ( 'NONE',  ( 7.703719777548943412E-34, -1.479221584281240009E-31, 1.000000000000000000 ) ) ;
#62725=ORIENTED_EDGE ( 'NONE', *, *, #27211, .T. ) ;
#62735=FACE_OUTER_BOUND ( 'NONE', #21926, .T. ) ;
#62755=PLANE ( 'NONE',  #6852 ) ;
#62780=CARTESIAN_POINT ( 'NONE',  ( -447.6627218934913230, 1.665334536937734811E-13, 83.55029585798817493 ) ) ;
#62794=DIRECTION ( 'NONE',  ( -1.110223024625156540E-16, -1.358505038629840220E-33, -1.000000000000000000 ) ) ;
#62807=SURFACE_SIDE_STYLE ('',( #36072 ) ) ;
#62818=ORIENTED_EDGE ( 'NONE', *, *, #2053, .T. ) ;
#62830=ORIENTED_EDGE ( 'NONE', *, *, #57352, .T. ) ;
#62849=CIRCLE ( 'NONE', #32506, 5.000000000000115463 ) ;
#62856=DIRECTION ( 'NONE',  ( 0.000000000000000000, 0.000000000000000000, -1.000000000000000000 ) ) ;
#62880=LINE ( 'NONE', #14681, #51743 ) ;
#62882=DIRECTION ( 'NONE',  ( 4.640644490319818793E-15, 1.000000000000000000, -7.216449660063517513E-16 ) ) ;
#62896=DIRECTION ( 'NONE',  ( -1.110223024625155594E-14, 0.000000000000000000, -1.000000000000000000 ) ) ;
#62941=PLANE ( 'NONE',  #31665 ) ;
#62970=DIRECTION ( 'NONE',  ( -1.387778780781445429E-16, 1.000000000000000000, 3.081487911019577365E-33 ) ) ;
#62979=EDGE_LOOP ( 'NONE', ( #3100, #32460, #43351, #64700, #12320, #52851, #50815 ) ) ;
#63046=ORIENTED_EDGE ( 'NONE', *, *, #64477, .T. ) ;
#63053=FILL_AREA_STYLE_COLOUR ( '', #64195 ) ;
#63076=CARTESIAN_POINT ( 'NONE',  ( -430.1627218934917209, 400.0000000000021600, 91.05029585799256608 ) ) ;
#63079=LINE ( 'NONE', #3304, #1838 ) ;
#63097=ORIENTED_EDGE ( 'NONE', *, *, #33944, .F. ) ;
#63123=ORIENTED_EDGE ( 'NONE', *, *, #53399, .T. ) ;
#63158=CLOSED_SHELL ( 'NONE', ( #57169, #37380, #55155, #57810, #31158, #6662, #768, #45961, #26923 ) ) ;
#63160=EDGE_CURVE ( 'NONE', #4775, #13320, #23757, .T. ) ;
#63199=VECTOR ( 'NONE', #68171, 1000.000000000000000 ) ;
#63242=EDGE_CURVE ( 'NONE', #6906, #32464, #60515, .T. ) ;
#63295=AXIS2_PLACEMENT_3D ( 'NONE', #7645, #49125, #966 ) ;
#63319=ORIENTED_EDGE ( 'NONE', *, *, #48649, .T. ) ;
#63326=VERTEX_POINT ( 'NONE', #69501 ) ;
#63327=CARTESIAN_POINT ( 'NONE',  ( -452.6627218934913230, 399.9999999999997726, 113.5502958579881891 ) ) ;
#63329=ORIENTED_EDGE ( 'NONE', *, *, #46004, .T. ) ;
#63359=DIRECTION ( 'NONE',  ( 8.893845946170152056E-21, -1.110223024625156294E-16, 1.000000000000000000 ) ) ;
#63365=DIRECTION ( 'NONE',  ( 7.703719777548945123E-34, 1.479221584281240009E-31, -1.000000000000000000 ) ) ;
#63368=EDGE_CURVE ( 'NONE', #46924, #50931, #12331, .T. ) ;
#63377=CARTESIAN_POINT ( 'NONE',  ( -444.3843108123961088, 394.6949978562683441, -128.2300613526361701 ) ) ;
#63384=STYLED_ITEM ( 'NONE', ( #31154 ), #40361 ) ;
#63390=CARTESIAN_POINT ( 'NONE',  ( 447.3372781065086201, 400.0000000000044338, 113.5502958579838122 ) ) ;
#63430=CARTESIAN_POINT ( 'NONE',  ( -417.6627218934915504, 399.9999999999957367, 78.55029585799222502 ) ) ;
#63434=FACE_OUTER_BOUND ( 'NONE', #41515, .T. ) ;
#63458=DIRECTION ( 'NONE',  ( -1.850169831522831466E-16, 1.000000000000000000, 1.110223024625156294E-16 ) ) ;
#63468=ORIENTED_EDGE ( 'NONE', *, *, #36224, .F. ) ;
#63486=AXIS2_PLACEMENT_3D ( 'NONE', #33559, #28618, #22991 ) ;
#63489=LINE ( 'NONE', #15303, #49426 ) ;
#63498=CARTESIAN_POINT ( 'NONE',  ( 447.3372781065085633, 399.9999999999998863, 113.5502958579882034 ) ) ;
#63528=DIRECTION ( 'NONE',  ( 1.387778780781445429E-16, -1.000000000000000000, -3.081487911019577365E-33 ) ) ;
#63544=CARTESIAN_POINT ( 'NONE',  ( 429.8372781065087338, 388.0000000000065938, 96.05029585798857283 ) ) ;
#63553=CARTESIAN_POINT ( 'NONE',  ( -452.6627218934913230, 177.8591479523843475, -111.4497041420117966 ) ) ;
#63557=CARTESIAN_POINT ( 'NONE',  ( 433.3728120124415568, 395.0000000000001137, -132.4852380479447902 ) ) ;
#63592=DIRECTION ( 'NONE',  ( -1.000000000000000000, -1.387778780781445676E-16, 0.000000000000000000 ) ) ;
#63616=EDGE_CURVE ( 'NONE', #23082, #40754, #25848, .T. ) ;
#63708=CARTESIAN_POINT ( 'NONE',  ( 112.3013380801408800, 395.0000000000065938, -128.9497041420121093 ) ) ;
#63726=APPLICATION_CONTEXT ( 'automotive_design' ) ;
#63735=FACE_OUTER_BOUND ( 'NONE', #36991, .T. ) ;
#63752=PLANE ( 'NONE',  #10270 ) ;
#63754=DIRECTION ( 'NONE',  ( 1.000000000000000000, 1.001918829714556097E-14, -9.899279560275163638E-15 ) ) ;
#63787=DIRECTION ( 'NONE',  ( 1.387778780781445429E-16, -1.000000000000000000, -3.081487911019577365E-33 ) ) ;
#63791=DIRECTION ( 'NONE',  ( -1.000000000000000000, 0.000000000000000000, 0.000000000000000000 ) ) ;
#63794=ORIENTED_EDGE ( 'NONE', *, *, #65532, .T. ) ;
#63814=ORIENTED_EDGE ( 'NONE', *, *, #34434, .T. ) ;
#63820=CIRCLE ( 'NONE', #66057, 5.000000000000004441 ) ;
#63831=EDGE_CURVE ( 'NONE', #55220, #45879, #27922, .T. ) ;
#63846=MANIFOLD_SOLID_BREP ( 'Cut-Extrude1[4]', #8076 ) ;
#63854=DIRECTION ( 'NONE',  ( -0.7071067811865473507, -1.232595164407830946E-32, 0.7071067811865476838 ) ) ;
#63860=VERTEX_POINT ( 'NONE', #18671 ) ;
#63875=DIRECTION ( 'NONE',  ( 1.000000000000000000, 1.387778780781445429E-16, 0.000000000000000000 ) ) ;
#63883=VERTEX_POINT ( 'NONE', #61232 ) ;
#63885=DIRECTION ( 'NONE',  ( -1.000000000000000000, 0.000000000000000000, 0.000000000000000000 ) ) ;
#63891=CARTESIAN_POINT ( 'NONE',  ( 312.3372781065084496, 394.9999999999999432, -21.44970414201177888 ) ) ;
#63892=VERTEX_POINT ( 'NONE', #24303 ) ;
#63947=EDGE_LOOP ( 'NONE', ( #50899, #36164, #31355, #648 ) ) ;
#64008=CARTESIAN_POINT ( 'NONE',  ( -417.6627218934913230, 219.4906275429376308, -144.4497041420118819 ) ) ;
#64053=CARTESIAN_POINT ( 'NONE',  ( -444.4229916354184411, 394.6798985497180752, 96.40978294693171335 ) ) ;
#64062=MANIFOLD_SOLID_BREP ( 'Angle iron 35 X 35 X 5(3)', #63158 ) ;
#64072=ADVANCED_FACE ( 'NONE', ( #1010 ), #28079, .F. ) ;
#64079=ORIENTED_EDGE ( 'NONE', *, *, #65508, .F. ) ;
#64080=ADVANCED_FACE ( 'NONE', ( #38642 ), #59728, .T. ) ;
#64082=ORIENTED_EDGE ( 'NONE', *, *, #12077, .T. ) ;
#64085=FILL_AREA_STYLE ('',( #63053 ) ) ;
#64099=PRODUCT_DEFINITION_CONTEXT ( 'detailed design', #33228, 'design' ) ;
#64120=CYLINDRICAL_SURFACE ( 'NONE', #10847, 5.000000000000004441 ) ;
#64136=AXIS2_PLACEMENT_3D ( 'NONE', #29354, #67350, #40257 ) ;
#64146=CARTESIAN_POINT ( 'NONE',  ( -447.6627218934919483, 370.0000000000064233, -141.4497041420121661 ) ) ;
#64151=CARTESIAN_POINT ( 'NONE',  ( 112.3013380801408658, 388.0000000000065938, -123.9497041420121235 ) ) ;
#64167=CARTESIAN_POINT ( 'NONE',  ( 50.98853755884153571, 388.0000000000071054, 101.0502958579881465 ) ) ;
#64175=MANIFOLD_SOLID_BREP ( 'Cut-Extrude1[2]', #22676 ) ;
#64195=COLOUR_RGB ( '',0.7921568627450980005, 0.8196078431372548767, 0.9333333333333333481 ) ;
#64218=ORIENTED_EDGE ( 'NONE', *, *, #17361, .F. ) ;
#64221=EDGE_CURVE ( 'NONE', #1580, #20970, #60562, .T. ) ;
#64225=DIRECTION ( 'NONE',  ( 1.387778780781446169E-16, -1.000000000000000000, -3.469446951953615421E-17 ) ) ;
#64233=CARTESIAN_POINT ( 'NONE',  ( 440.2662102946433151, 395.0000000000066507, -139.3786363301462927 ) ) ;
#64259=ORIENTED_EDGE ( 'NONE', *, *, #46703, .T. ) ;
#64275=ADVANCED_BREP_SHAPE_REPRESENTATION ( '', ( #40140, #64062, #16744, #16860, #40361, #41747, #40938, #16524, #40015, #64175, #17808, #63846, #66832 ), #12890 ) ;
#64312=EDGE_LOOP ( 'NONE', ( #19839, #61962, #10262, #33782 ) ) ;
#64317=ORIENTED_EDGE ( 'NONE', *, *, #67684, .F. ) ;
#64330=PLANE ( 'NONE',  #14222 ) ;
#64366=COLOUR_RGB ( '',0.7921568627450980005, 0.8196078431372548767, 0.9333333333333333481 ) ;
#64445=ORIENTED_EDGE ( 'NONE', *, *, #14230, .F. ) ;
#64476=ORIENTED_EDGE ( 'NONE', *, *, #2955, .F. ) ;
#64477=EDGE_CURVE ( 'NONE', #7875, #8973, #17885, .T. ) ;
#64482=CARTESIAN_POINT ( 'NONE',  ( -417.6627218934913230, 179.4906275429376308, -144.4497041420118819 ) ) ;
#64485=DIRECTION ( 'NONE',  ( 1.000000000000000000, 1.132072239499580971E-16, -1.697513318603925187E-16 ) ) ;
#64500=ORIENTED_EDGE ( 'NONE', *, *, #31403, .F. ) ;
#64521=VERTEX_POINT ( 'NONE', #32293 ) ;
#64529=CARTESIAN_POINT ( 'NONE',  ( 50.98853755884157124, 395.0000000000065938, -128.9497041420121946 ) ) ;
#64537=CARTESIAN_POINT ( 'NONE',  ( -444.1138056043201914, 394.7873829578389859, -130.7180718971919475 ) ) ;
#64538=AXIS2_PLACEMENT_3D ( 'NONE', #34366, #44187, #66725 ) ;
#64543=EDGE_CURVE ( 'NONE', #32531, #37758, #7825, .T. ) ;
#64586=CARTESIAN_POINT ( 'NONE',  ( -442.6627218934914367, 399.9999999999998863, -136.4497041420118251 ) ) ;
#64605=CARTESIAN_POINT ( 'NONE',  ( 412.3372781065085633, 219.4906275429376308, -144.4497041420117682 ) ) ;
#64619=DIRECTION ( 'NONE',  ( 1.000000000000000000, 0.000000000000000000, 0.000000000000000000 ) ) ;
#64621=CARTESIAN_POINT ( 'NONE',  ( 445.3372781065085633, 217.8591479523844612, -111.4497041420119388 ) ) ;
#64642=LINE ( 'NONE', #11499, #22132 ) ;
#64689=CARTESIAN_POINT ( 'NONE',  ( -444.4229916354184411, 388.0000000000064801, -128.9497041420121093 ) ) ;
#64700=ORIENTED_EDGE ( 'NONE', *, *, #18798, .T. ) ;
#64723=FACE_OUTER_BOUND ( 'NONE', #66784, .T. ) ;
#64739=VECTOR ( 'NONE', #36223, 1000.000000000000000 ) ;
#64741=ORIENTED_EDGE ( 'NONE', *, *, #23968, .T. ) ;
#64746=DIRECTION ( 'NONE',  ( 1.000000000000000000, 0.000000000000000000, 0.000000000000000000 ) ) ;
#64773=ORIENTED_EDGE ( 'NONE', *, *, #29125, .T. ) ;
#64822=FACE_OUTER_BOUND ( 'NONE', #16663, .T. ) ;
#64836=CARTESIAN_POINT ( 'NONE',  ( -452.6627218934860366, 395.0000000000064801, -123.9497041420119530 ) ) ;
#64840=AXIS2_PLACEMENT_3D ( 'NONE', #12433, #28613, #34601 ) ;
#64860=LINE ( 'NONE', #49353, #32913 ) ;
#64873=ORIENTED_EDGE ( 'NONE', *, *, #47873, .T. ) ;
#64877=DIRECTION ( 'NONE',  ( -0.7071067811865476838, 0.000000000000000000, -0.7071067811865474617 ) ) ;
#64890=FACE_OUTER_BOUND ( 'NONE', #48795, .T. ) ;
#64905=EDGE_CURVE ( 'NONE', #8003, #59605, #65248, .T. ) ;
#64906=ORIENTED_EDGE ( 'NONE', *, *, #17130, .T. ) ;
#64908=ADVANCED_FACE ( 'NONE', ( #66321 ), #6146, .F. ) ;
#64936=ORIENTED_EDGE ( 'NONE', *, *, #5952, .F. ) ;
#64980=CARTESIAN_POINT ( 'NONE',  ( 429.8372781065087338, 394.9999999999999432, 96.05029585798857283 ) ) ;
#64984=ORIENTED_EDGE ( 'NONE', *, *, #66260, .F. ) ;
#64986=DIRECTION ( 'NONE',  ( -4.270088556250601699E-16, -0.000000000000000000, -1.000000000000000000 ) ) ;
#65027=AXIS2_PLACEMENT_3D ( 'NONE', #27778, #11585, #10207 ) ;
#65029=DIRECTION ( 'NONE',  ( -2.922263668027335568E-20, -1.000000000000000000, -1.110223024625156294E-16 ) ) ;
#65039=EDGE_CURVE ( 'NONE', #15022, #21328, #20146, .T. ) ;
#65042=EDGE_CURVE ( 'NONE', #52163, #6017, #7804, .T. ) ;
#65046=DIRECTION ( 'NONE',  ( 1.000000000000000000, 1.387778780781448634E-16, -1.387778780781445676E-15 ) ) ;
#65059=FILL_AREA_STYLE_COLOUR ( '', #4691 ) ;
#65088=CARTESIAN_POINT ( 'NONE',  ( 412.3372781065086201, 399.9999999999998863, 113.5502958579881891 ) ) ;
#65098=CARTESIAN_POINT ( 'NONE',  ( -442.6627218934912662, 394.9999999999998295, 99.85872701201111568 ) ) ;
#65104=DIRECTION ( 'NONE',  ( -1.850371928290090422E-16, 1.000000000000000000, 1.110223024625156171E-16 ) ) ;
#65108=ORIENTED_EDGE ( 'NONE', *, *, #21582, .T. ) ;
#65109=EDGE_CURVE ( 'NONE', #4775, #32147, #51164, .T. ) ;
#65128=CARTESIAN_POINT ( 'NONE',  ( -444.2277112916228816, 394.7494927581580555, 94.61947695070884379 ) ) ;
#65145=CARTESIAN_POINT ( 'NONE',  ( 447.3372781065086201, 0.000000000000000000, 113.5502958579881749 ) ) ;
#65248=LINE ( 'NONE', #22684, #43716 ) ;
#65262=DIRECTION ( 'NONE',  ( -1.000000000000000000, -1.001918046209079887E-14, 9.729495617646301779E-15 ) ) ;
#65265=VERTEX_POINT ( 'NONE', #58836 ) ;
#65266=ADVANCED_FACE ( 'NONE', ( #53553 ), #42327, .T. ) ;
#65340=( BOUNDED_CURVE ( )  B_SPLINE_CURVE ( 3, ( #23736, #56788, #13189, #2624 ),
 .UNSPECIFIED., .F., .F. ) 
 B_SPLINE_CURVE_WITH_KNOTS ( ( 4, 4 ),
 ( -2.664535259100375697E-15, 1.570796326794896558 ),
 .UNSPECIFIED. ) 
 CURVE ( )  GEOMETRIC_REPRESENTATION_ITEM ( )  RATIONAL_B_SPLINE_CURVE ( ( 1.000000000000000000, 0.8047378541243643824, 0.8047378541243643824, 1.000000000000000000 ) ) 
 REPRESENTATION_ITEM ( '' )  );
#65351=ORIENTED_EDGE ( 'NONE', *, *, #28519, .T. ) ;
#65355=VERTEX_POINT ( 'NONE', #6059 ) ;
#65382=DIRECTION ( 'NONE',  ( -1.000000000000000000, -1.110223024625155594E-14, 1.110223024625155594E-14 ) ) ;
#65402=CARTESIAN_POINT ( 'NONE',  ( 442.3372781065085633, 370.0000000000001137, -146.4497041420116830 ) ) ;
#65427=ORIENTED_EDGE ( 'NONE', *, *, #67681, .T. ) ;
#65433=ORIENTED_EDGE ( 'NONE', *, *, #8681, .T. ) ;
#65439=EDGE_LOOP ( 'NONE', ( #40065, #24572, #57578, #2180 ) ) ;
#65456=CIRCLE ( 'NONE', #10563, 5.000000000000170530 ) ;
#65466=SURFACE_SIDE_STYLE ('',( #54182 ) ) ;
#65495=MECHANICAL_DESIGN_GEOMETRIC_PRESENTATION_REPRESENTATION('',(#40936),#65648);
#65502=VECTOR ( 'NONE', #30870, 1000.000000000000000 ) ;
#65508=EDGE_CURVE ( 'NONE', #23473, #24241, #24353, .T. ) ;
#65516=AXIS2_PLACEMENT_3D ( 'NONE', #42712, #37432, #499 ) ;
#65523=CARTESIAN_POINT ( 'NONE',  ( -452.6627218934913799, 399.9999999999953957, 113.5502958579925803 ) ) ;
#65532=EDGE_CURVE ( 'NONE', #21613, #9937, #983, .T. ) ;
#65563=DIRECTION ( 'NONE',  ( 0.000000000000000000, 0.000000000000000000, 1.000000000000000000 ) ) ;
#65568=CIRCLE ( 'NONE', #423, 5.000000000000004441 ) ;
#65580=DIRECTION ( 'NONE',  ( -1.020422603260505347E-14, 1.000000000000000000, 5.551115123125782702E-17 ) ) ;
#65619=ORIENTED_EDGE ( 'NONE', *, *, #24554, .T. ) ;
#65635=ORIENTED_EDGE ( 'NONE', *, *, #48500, .F. ) ;
#65638=DIRECTION ( 'NONE',  ( 0.7071067811865476838, -5.551115123125782086E-17, 0.7071067811865473507 ) ) ;
#65640=CARTESIAN_POINT ( 'NONE',  ( -447.6627218934914367, 389.9999999999954525, 108.5502958579925235 ) ) ;
#65648=( GEOMETRIC_REPRESENTATION_CONTEXT ( 3 ) GLOBAL_UNCERTAINTY_ASSIGNED_CONTEXT ( ( #36693 ) ) GLOBAL_UNIT_ASSIGNED_CONTEXT ( ( #37192, #26309, #10119 ) ) REPRESENTATION_CONTEXT ( 'NONE', 'WORKASPACE' ) );
#65653=VECTOR ( 'NONE', #28462, 1000.000000000000000 ) ;
#65665=ADVANCED_FACE ( 'NONE', ( #26416 ), #57736, .T. ) ;
#65694=DIRECTION ( 'NONE',  ( 1.697742017499683849E-16, -1.665334536937734564E-16, 1.000000000000000000 ) ) ;
#65704=DIRECTION ( 'NONE',  ( 1.000000000000000000, 1.748373411921809651E-16, 2.371692252312040348E-20 ) ) ;
#65706=EDGE_CURVE ( 'NONE', #67714, #15124, #26958, .T. ) ;
#65708=VECTOR ( 'NONE', #40579, 1000.000000000000000 ) ;
#65711=CIRCLE ( 'NONE', #47698, 5.000000000000004441 ) ;
#65723=LINE ( 'NONE', #28065, #261 ) ;
#65732=EDGE_LOOP ( 'NONE', ( #54349, #53578, #742, #37252, #20914, #66519, #19668, #28056, #45073, #56387, #15184, #30880, #47939, #42086, #36893 ) ) ;
#65733=CARTESIAN_POINT ( 'NONE',  ( 429.8372781065086201, 395.0000000000042633, 101.0502958579843806 ) ) ;
#65734=PLANE ( 'NONE',  #51137 ) ;
#65758=ORIENTED_EDGE ( 'NONE', *, *, #37086, .F. ) ;
#65792=LINE ( 'NONE', #28132, #29597 ) ;
#65803=CARTESIAN_POINT ( 'NONE',  ( 444.4083459183741525, 365.0000000000000000, 110.6213636698541336 ) ) ;
#65827=B_SPLINE_CURVE_WITH_KNOTS ( 'NONE', 3,
 ( #35260, #61981, #46151, #9570, #20452, #67976, #8538, #63377, #9220, #29984 ),
 .UNSPECIFIED., .F., .F.,
 ( 4, 2, 2, 2, 4 ),
 ( 0.000000000000000000, 0.001080786818375923915, 0.002161573636751847830, 0.003242360455127771962, 0.004323147273503695660 ),
 .UNSPECIFIED. ) ;
#65831=CARTESIAN_POINT ( 'NONE',  ( -422.6627218934914936, 399.9999999999998863, -141.4497041420118535 ) ) ;
#65832=DIRECTION ( 'NONE',  ( -0.7071067811865475727, 0.000000000000000000, -0.7071067811865474617 ) ) ;
#65839=DIRECTION ( 'NONE',  ( -9.115745035929406798E-64, 3.469446951953612956E-17, -1.000000000000000000 ) ) ;
#65877=LINE ( 'NONE', #13095, #8703 ) ;
#65927=VECTOR ( 'NONE', #25671, 1000.000000000000000 ) ;
#65968=LINE ( 'NONE', #31612, #9569 ) ;
#65972=ORIENTED_EDGE ( 'NONE', *, *, #61391, .T. ) ;
#65991=ORIENTED_EDGE ( 'NONE', *, *, #24880, .T. ) ;
#65998=DIRECTION ( 'NONE',  ( 0.000000000000000000, -3.469446951953614805E-17, 1.000000000000000000 ) ) ;
#66057=AXIS2_PLACEMENT_3D ( 'NONE', #3224, #67940, #8849 ) ;
#66079=LINE ( 'NONE', #11526, #50940 ) ;
#66092=CARTESIAN_POINT ( 'NONE',  ( 50.98853755884140071, 400.0000000000071054, 101.0502958579881465 ) ) ;
#66103=AXIS2_PLACEMENT_3D ( 'NONE', #18194, #65694, #39303 ) ;
#66111=AXIS2_PLACEMENT_3D ( 'NONE', #19311, #8426, #34814 ) ;
#66112=PLANE ( 'NONE',  #8435 ) ;
#66113=DIRECTION ( 'NONE',  ( 1.387778780781445922E-16, -1.000000000000000000, -1.232595164407830946E-32 ) ) ;
#66116=CARTESIAN_POINT ( 'NONE',  ( 437.3372781065084496, 395.0000000000043201, 103.5502958579839259 ) ) ;
#66142=PLANE ( 'NONE',  #25936 ) ;
#66153=EDGE_CURVE ( 'NONE', #38085, #63883, #1591, .T. ) ;
#66162=CARTESIAN_POINT ( 'NONE',  ( -452.6627218934914367, 399.9999999999998863, -116.4497041420118393 ) ) ;
#66201=LINE ( 'NONE', #23958, #38977 ) ;
#66202=VECTOR ( 'NONE', #26612, 1000.000000000000000 ) ;
#66226=EDGE_LOOP ( 'NONE', ( #66711, #67935, #33167, #34035 ) ) ;
#66259=VECTOR ( 'NONE', #22272, 1000.000000000000000 ) ;
#66260=EDGE_CURVE ( 'NONE', #55579, #366, #46229, .T. ) ;
#66267=EDGE_LOOP ( 'NONE', ( #5872, #65108, #55141, #38880, #49400, #11625, #14606 ) ) ;
#66280=ORIENTED_EDGE ( 'NONE', *, *, #20089, .T. ) ;
#66292=EDGE_LOOP ( 'NONE', ( #62063, #43240, #15568, #3963 ) ) ;
#66297=DIRECTION ( 'NONE',  ( -1.000000000000000000, 0.000000000000000000, 0.000000000000000000 ) ) ;
#66320=ORIENTED_EDGE ( 'NONE', *, *, #534, .T. ) ;
#66321=FACE_OUTER_BOUND ( 'NONE', #33059, .T. ) ;
#66339=ORIENTED_EDGE ( 'NONE', *, *, #27009, .F. ) ;
#66346=CARTESIAN_POINT ( 'NONE',  ( 414.4083459183745504, 395.0000000000065938, -113.5207719538776843 ) ) ;
#66359=CARTESIAN_POINT ( 'NONE',  ( -417.6627218934913230, 179.4906275429376308, -144.4497041420118819 ) ) ;
#66360=ORIENTED_EDGE ( 'NONE', *, *, #49927, .F. ) ;
#66391=DIRECTION ( 'NONE',  ( -1.020422603260505347E-14, 1.000000000000000000, 5.551115123125782702E-17 ) ) ;
#66400=EDGE_CURVE ( 'NONE', #45368, #23473, #33869, .T. ) ;
#66412=CARTESIAN_POINT ( 'NONE',  ( 412.3372781065085633, 179.4906275429376024, -146.4497041420117682 ) ) ;
#66422=ADVANCED_FACE ( 'NONE', ( #68310 ), #56022, .T. ) ;
#66443=VECTOR ( 'NONE', #45571, 1000.000000000000000 ) ;
#66459=CARTESIAN_POINT ( 'NONE',  ( 442.3372781065084496, 390.0000000000043201, 108.5502958579838690 ) ) ;
#66475=LINE ( 'NONE', #22845, #35722 ) ;
#66478=DIRECTION ( 'NONE',  ( 1.000000000000000000, 2.465190328815661345E-32, 0.000000000000000000 ) ) ;
#66488=ORIENTED_EDGE ( 'NONE', *, *, #36205, .T. ) ;
#66491=LINE ( 'NONE', #39739, #20707 ) ;
#66519=ORIENTED_EDGE ( 'NONE', *, *, #34022, .T. ) ;
#66523=( NAMED_UNIT ( * ) PLANE_ANGLE_UNIT ( ) SI_UNIT ( $, .RADIAN. ) );
#66548=VERTEX_POINT ( 'NONE', #3251 ) ;
#66562=CARTESIAN_POINT ( 'NONE',  ( 424.8372781065089612, 400.0000000000066507, 91.05029585798857283 ) ) ;
#66593=VERTEX_POINT ( 'NONE', #5642 ) ;
#66617=CARTESIAN_POINT ( 'NONE',  ( -439.4229916354183274, 394.9999999999998295, 96.05029585798874336 ) ) ;
#66633=CARTESIAN_POINT ( 'NONE',  ( -445.5916540816260749, 394.9999999999953957, 106.4792280461270479 ) ) ;
#66637=PLANE ( 'NONE',  #50317 ) ;
#66643=DIRECTION ( 'NONE',  ( 0.000000000000000000, 6.405132834375902056E-16, -1.000000000000000000 ) ) ;
#66653=CYLINDRICAL_SURFACE ( 'NONE', #58597, 5.000000000000004441 ) ;
#66711=ORIENTED_EDGE ( 'NONE', *, *, #13298, .T. ) ;
#66717=CARTESIAN_POINT ( 'NONE',  ( -452.6627218934860366, 395.0000000000064801, -123.9497041420121235 ) ) ;
#66725=DIRECTION ( 'NONE',  ( 1.000000000000000000, 0.000000000000000000, 0.000000000000000000 ) ) ;
#66740=VERTEX_POINT ( 'NONE', #51357 ) ;
#66784=EDGE_LOOP ( 'NONE', ( #42246, #31327, #55881, #61636 ) ) ;
#66805=SURFACE_STYLE_USAGE ( .BOTH. , #61160 ) ;
#66811=CARTESIAN_POINT ( 'NONE',  ( -430.1627218934916073, 394.9999999999998295, 91.05029585798840230 ) ) ;
#66824=ORIENTED_EDGE ( 'NONE', *, *, #38999, .F. ) ;
#66826=ORIENTED_EDGE ( 'NONE', *, *, #37636, .T. ) ;
#66832=AXIS2_PLACEMENT_3D ( 'NONE', #50530, #44558, #8319 ) ;
#66845=VERTEX_POINT ( 'NONE', #29203 ) ;
#66865=ORIENTED_EDGE ( 'NONE', *, *, #59715, .F. ) ;
#66869=VECTOR ( 'NONE', #299, 1000.000000000000000 ) ;
#66895=CARTESIAN_POINT ( 'NONE',  ( -439.4229916354183274, 388.0000000000064801, -123.9497041420119530 ) ) ;
#66900=DIRECTION ( 'NONE',  ( -0.7071067811865474617, 0.000000000000000000, 0.7071067811865474617 ) ) ;
#66941=ADVANCED_FACE ( 'NONE', ( #5228 ), #62941, .T. ) ;
#66962=ORIENTED_EDGE ( 'NONE', *, *, #69547, .T. ) ;
#66972=EDGE_CURVE ( 'NONE', #13791, #4404, #10845, .T. ) ;
#66974=VECTOR ( 'NONE', #63365, 1000.000000000000000 ) ;
#66989=DIRECTION ( 'NONE',  ( 1.000000000000000000, 0.000000000000000000, 0.000000000000000000 ) ) ;
#67019=VECTOR ( 'NONE', #11572, 1000.000000000000114 ) ;
#67079=( LENGTH_UNIT ( ) NAMED_UNIT ( * ) SI_UNIT ( .MILLI., .METRE. ) );
#67094=CARTESIAN_POINT ( 'NONE',  ( 447.3372781065084496, 390.0000000000043769, 103.5502958579838264 ) ) ;
#67121=ORIENTED_EDGE ( 'NONE', *, *, #4617, .F. ) ;
#67127=AXIS2_PLACEMENT_3D ( 'NONE', #16154, #49188, #22477 ) ;
#67154=LINE ( 'NONE', #2765, #30465 ) ;
#67156=LINE ( 'NONE', #3804, #16517 ) ;
#67160=CIRCLE ( 'NONE', #13269, 5.000000000000170530 ) ;
#67170=CARTESIAN_POINT ( 'NONE',  ( 447.3372781065085633, 395.0000000000043769, 101.0502958579842101 ) ) ;
#67172=VECTOR ( 'NONE', #28370, 1000.000000000000000 ) ;
#67182=CARTESIAN_POINT ( 'NONE',  ( 424.8372781065088475, 394.9999999999999432, 91.05029585798857283 ) ) ;
#67198=EDGE_CURVE ( 'NONE', #55194, #38457, #66079, .T. ) ;
#67209=( BOUNDED_CURVE ( )  B_SPLINE_CURVE ( 3, ( #27452, #48203, #10239, #58425 ),
 .UNSPECIFIED., .F., .F. ) 
 B_SPLINE_CURVE_WITH_KNOTS ( ( 4, 4 ),
 ( 1.570796326794874131, 3.141592653589778461 ),
 .UNSPECIFIED. ) 
 CURVE ( )  GEOMETRIC_REPRESENTATION_ITEM ( )  RATIONAL_B_SPLINE_CURVE ( ( 1.000000000000000000, 0.8047378541243631611, 0.8047378541243631611, 1.000000000000000000 ) ) 
 REPRESENTATION_ITEM ( '' )  );
#67230=LINE ( 'NONE', #28529, #18210 ) ;
#67241=DIRECTION ( 'NONE',  ( 0.000000000000000000, -7.395570986446983486E-32, -1.000000000000000000 ) ) ;
#67250=CARTESIAN_POINT ( 'NONE',  ( 442.3372781065089612, 370.0000000000065938, -141.4497041420121661 ) ) ;
#67281=CARTESIAN_POINT ( 'NONE',  ( -417.6627218934913230, 1.665334536937734811E-13, 113.5502958579881749 ) ) ;
#67290=ORIENTED_EDGE ( 'NONE', *, *, #47530, .F. ) ;
#67329=CARTESIAN_POINT ( 'NONE',  ( 447.3372781065086770, 400.0000000000000568, -146.4497041420117966 ) ) ;
#67332=DIRECTION ( 'NONE',  ( -1.000000000000000000, -1.387778780781446169E-16, 0.000000000000000000 ) ) ;
#67350=DIRECTION ( 'NONE',  ( -4.314083075427411048E-32, -1.000000000000000000, -6.123233995736763571E-17 ) ) ;
#67371=CARTESIAN_POINT ( 'NONE',  ( 447.3372781065085633, 395.0000000000043769, 101.0502958579842243 ) ) ;
#67374=ORIENTED_EDGE ( 'NONE', *, *, #49373, .F. ) ;
#67381=CARTESIAN_POINT ( 'NONE',  ( 447.3372781065085064, 400.0000000000001137, -146.4497041420118535 ) ) ;
#67410=CARTESIAN_POINT ( 'NONE',  ( 447.3372781065085064, 395.0000000000043769, 103.5502958579838264 ) ) ;
#67412=DIRECTION ( 'NONE',  ( 1.000000000000000000, 0.000000000000000000, 0.000000000000000000 ) ) ;
#67421=CARTESIAN_POINT ( 'NONE',  ( 412.3372781065085633, 219.4906275429376308, 111.5502958579881749 ) ) ;
#67458=VERTEX_POINT ( 'NONE', #1882 ) ;
#67490=EDGE_LOOP ( 'NONE', ( #30980, #53245, #16871, #69475 ) ) ;
#67499=EDGE_CURVE ( 'NONE', #67779, #60980, #18047, .T. ) ;
#67509=DIRECTION ( 'NONE',  ( -1.000000000000000000, -1.387778780781445922E-16, 0.000000000000000000 ) ) ;
#67553=DIRECTION ( 'NONE',  ( -0.000000000000000000, 1.000000000000000000, -0.000000000000000000 ) ) ;
#67555=DIRECTION ( 'NONE',  ( 1.000000000000000000, -1.232595164407830946E-32, -7.703719777548943412E-34 ) ) ;
#67573=ORIENTED_EDGE ( 'NONE', *, *, #67499, .T. ) ;
#67580=EDGE_CURVE ( 'NONE', #60980, #7875, #45402, .T. ) ;
#67596=LINE ( 'NONE', #40854, #14320 ) ;
#67606=( BOUNDED_CURVE ( )  B_SPLINE_CURVE ( 3, ( #3703, #24822, #57866, #20227 ),
 .UNSPECIFIED., .F., .F. ) 
 B_SPLINE_CURVE_WITH_KNOTS ( ( 4, 4 ),
 ( -8.881784197001252323E-16, 1.570796326794886344 ),
 .UNSPECIFIED. ) 
 CURVE ( )  GEOMETRIC_REPRESENTATION_ITEM ( )  RATIONAL_B_SPLINE_CURVE ( ( 1.000000000000000000, 0.8047378541243671579, 0.8047378541243671579, 1.000000000000000000 ) ) 
 REPRESENTATION_ITEM ( '' )  );
#67622=STYLED_ITEM ( 'NONE', ( #59072 ), #17808 ) ;
#67631=CLOSED_SHELL ( 'NONE', ( #52164, #66422, #24102, #3116, #44603, #34960, #18100, #10536, #2487, #14923, #3632, #12408, #12414, #65665, #24412, #45742, #33024, #48858, #57490, #68757 ) ) ;
#67668=VECTOR ( 'NONE', #51261, 1000.000000000000000 ) ;
#67681=EDGE_CURVE ( 'NONE', #54939, #48080, #9854, .T. ) ;
#67684=EDGE_CURVE ( 'NONE', #20962, #66740, #15126, .T. ) ;
#67685=DIRECTION ( 'NONE',  ( -1.000000000000000000, 0.000000000000000000, 0.000000000000000000 ) ) ;
#67704=DIRECTION ( 'NONE',  ( 0.000000000000000000, 1.000000000000000000, -1.479221584281239571E-31 ) ) ;
#67713=CARTESIAN_POINT ( 'NONE',  ( 447.3372781065084496, 399.9999999999998863, 113.5502958579881465 ) ) ;
#67714=VERTEX_POINT ( 'NONE', #68917 ) ;
#67744=CARTESIAN_POINT ( 'NONE',  ( 442.3372781065085633, 400.0000000000000568, -116.4497041420118393 ) ) ;
#67763=ADVANCED_FACE ( 'NONE', ( #57006 ), #52738, .F. ) ;
#67777=VECTOR ( 'NONE', #22584, 1000.000000000000000 ) ;
#67779=VERTEX_POINT ( 'NONE', #42202 ) ;
#67785=VECTOR ( 'NONE', #58206, 1000.000000000000000 ) ;
#67808=COLOUR_RGB ( '',0.7921568627450980005, 0.8196078431372548767, 0.9333333333333333481 ) ;
#67811=DIRECTION ( 'NONE',  ( 1.110223024625156294E-16, 0.000000000000000000, -1.000000000000000000 ) ) ;
#67826=VECTOR ( 'NONE', #55215, 1000.000000000000000 ) ;
#67862=CARTESIAN_POINT ( 'NONE',  ( 412.3372781065086201, 400.0000000000000568, -146.4497041420118251 ) ) ;
#67871=AXIS2_PLACEMENT_3D ( 'NONE', #35217, #4254, #37273 ) ;
#67890=EDGE_CURVE ( 'NONE', #13335, #63326, #6288, .T. ) ;
#67893=CARTESIAN_POINT ( 'NONE',  ( 442.3372781065085633, 367.0710678118655892, -141.4497041420118251 ) ) ;
#67933=VECTOR ( 'NONE', #24967, 1000.000000000000000 ) ;
#67935=ORIENTED_EDGE ( 'NONE', *, *, #15575, .T. ) ;
#67939=EDGE_LOOP ( 'NONE', ( #54407, #15360, #44559, #62434 ) ) ;
#67940=DIRECTION ( 'NONE',  ( 1.387778780781446169E-16, -1.000000000000000000, -3.469446951953615421E-17 ) ) ;
#67975=CIRCLE ( 'NONE', #572, 5.000000000000004441 ) ;
#67976=CARTESIAN_POINT ( 'NONE',  ( -444.1126562889745060, 394.7876926391177790, -127.1788437718730194 ) ) ;
#67988=EDGE_CURVE ( 'NONE', #21636, #12229, #34486, .T. ) ;
#67996=EDGE_CURVE ( 'NONE', #29979, #43634, #416, .T. ) ;
#67998=ORIENTED_EDGE ( 'NONE', *, *, #27891, .F. ) ;
#68014=AXIS2_PLACEMENT_3D ( 'NONE', #34514, #14078, #23257 ) ;
#68028=( BOUNDED_CURVE ( )  B_SPLINE_CURVE ( 3, ( #49592, #732, #1078, #7413 ),
 .UNSPECIFIED., .F., .F. ) 
 B_SPLINE_CURVE_WITH_KNOTS ( ( 4, 4 ),
 ( 1.570796326794902109, 3.141592653589793116 ),
 .UNSPECIFIED. ) 
 CURVE ( )  GEOMETRIC_REPRESENTATION_ITEM ( )  RATIONAL_B_SPLINE_CURVE ( ( 1.000000000000000000, 0.8047378541243662697, 0.8047378541243662697, 1.000000000000000000 ) ) 
 REPRESENTATION_ITEM ( '' )  );
#68059=AXIS2_PLACEMENT_3D ( 'NONE', #24290, #52391, #29544 ) ;
#68065=DIRECTION ( 'NONE',  ( 1.334402673828311663E-15, -1.000000000000000000, -1.974915957265903643E-15 ) ) ;
#68078=DIRECTION ( 'NONE',  ( -3.081487911019579554E-32, -1.000000000000000000, -3.469446951953612956E-17 ) ) ;
#68085=FACE_OUTER_BOUND ( 'NONE', #26615, .T. ) ;
#68089=DIRECTION ( 'NONE',  ( 0.7071067811865473507, 0.000000000000000000, -0.7071067811865477948 ) ) ;
#68123=CIRCLE ( 'NONE', #23167, 5.000000000000004441 ) ;
#68125=VERTEX_POINT ( 'NONE', #9770 ) ;
#68129=ORIENTED_EDGE ( 'NONE', *, *, #34434, .F. ) ;
#68138=LINE ( 'NONE', #36116, #40947 ) ;
#68154=AXIS2_PLACEMENT_3D ( 'NONE', #50937, #41075, #62535 ) ;
#68165=AXIS2_PLACEMENT_3D ( 'NONE', #51073, #46826, #9195 ) ;
#68171=DIRECTION ( 'NONE',  ( 1.000000000000000000, 1.748373411921809651E-16, 2.371692252312040348E-20 ) ) ;
#68209=ORIENTED_EDGE ( 'NONE', *, *, #60611, .T. ) ;
#68217=ORIENTED_EDGE ( 'NONE', *, *, #35755, .F. ) ;
#68242=CARTESIAN_POINT ( 'NONE',  ( -442.6627218934913230, 399.9999999999997726, 108.5502958579881891 ) ) ;
#68274=DIRECTION ( 'NONE',  ( 9.109522253334613014E-16, 1.000000000000000000, -3.889846672687432470E-31 ) ) ;
#68286=VERTEX_POINT ( 'NONE', #49453 ) ;
#68296=DIRECTION ( 'NONE',  ( -2.922263668027335568E-20, -1.000000000000000000, -1.110223024625156294E-16 ) ) ;
#68307=ORIENTED_EDGE ( 'NONE', *, *, #25971, .F. ) ;
#68309=EDGE_CURVE ( 'NONE', #22785, #8973, #28361, .T. ) ;
#68310=FACE_OUTER_BOUND ( 'NONE', #35110, .T. ) ;
#68321=VERTEX_POINT ( 'NONE', #23791 ) ;
#68326=DIRECTION ( 'NONE',  ( -1.000000000000000000, 9.109522253334599209E-16, 4.270088556250601699E-16 ) ) ;
#68342=DIRECTION ( 'NONE',  ( -3.081487911019579554E-32, -1.000000000000000000, -3.469446951953612956E-17 ) ) ;
#68343=FACE_OUTER_BOUND ( 'NONE', #51947, .T. ) ;
#68395=VERTEX_POINT ( 'NONE', #47904 ) ;
#68415=LINE ( 'NONE', #47623, #5020 ) ;
#68422=CARTESIAN_POINT ( 'NONE',  ( -417.6627218934913230, 179.4906275429376308, 111.5502958579881749 ) ) ;
#68432=CARTESIAN_POINT ( 'NONE',  ( 433.3728120124416705, 395.0000000000066507, -132.4852380479447618 ) ) ;
#68485=EDGE_CURVE ( 'NONE', #5635, #68321, #8305, .T. ) ;
#68562=VECTOR ( 'NONE', #49361, 1000.000000000000000 ) ;
#68565=ORIENTED_EDGE ( 'NONE', *, *, #63242, .T. ) ;
#68596=ORIENTED_EDGE ( 'NONE', *, *, #31403, .T. ) ;
#68598=CARTESIAN_POINT ( 'NONE',  ( -305.1627218934913230, 399.9999999999997726, 1.050295857988214898 ) ) ;
#68616=CIRCLE ( 'NONE', #30466, 5.000000000000115463 ) ;
#68627=DIRECTION ( 'NONE',  ( 1.000000000000000000, 0.000000000000000000, 0.000000000000000000 ) ) ;
#68668=SURFACE_STYLE_FILL_AREA ( #64085 ) ;
#68696=CARTESIAN_POINT ( 'NONE',  ( 417.3372781065086201, 399.9999999999998863, 113.5502958579881891 ) ) ;
#68707=VERTEX_POINT ( 'NONE', #14099 ) ;
#68728=ORIENTED_EDGE ( 'NONE', *, *, #11964, .F. ) ;
#68741=EDGE_LOOP ( 'NONE', ( #810, #21523, #27785, #57998, #58085, #59737, #26700 ) ) ;
#68757=ADVANCED_FACE ( 'NONE', ( #35559 ), #45412, .F. ) ;
#68802=VERTEX_POINT ( 'NONE', #35208 ) ;
#68809=VECTOR ( 'NONE', #43466, 1000.000000000000000 ) ;
#68819=ORIENTED_EDGE ( 'NONE', *, *, #53901, .F. ) ;
#68827=LINE ( 'NONE', #35807, #12643 ) ;
#68863=ORIENTED_EDGE ( 'NONE', *, *, #52250, .T. ) ;
#68864=CARTESIAN_POINT ( 'NONE',  ( -20.16272189348855903, 400.0000000000064801, 321.0502958579853043 ) ) ;
#68866=EDGE_CURVE ( 'NONE', #51645, #39831, #62642, .T. ) ;
#68894=EDGE_CURVE ( 'NONE', #29891, #59106, #36597, .T. ) ;
#68913=FACE_OUTER_BOUND ( 'NONE', #39653, .T. ) ;
#68916=ORIENTED_EDGE ( 'NONE', *, *, #30667, .F. ) ;
#68917=CARTESIAN_POINT ( 'NONE',  ( 112.3013380801408658, 395.0000000000065938, -123.9497041420121235 ) ) ;
#68936=DIRECTION ( 'NONE',  ( -1.000000000000000000, 9.109522253334613014E-16, 0.000000000000000000 ) ) ;
#68983=EDGE_CURVE ( 'NONE', #63892, #32531, #11562, .T. ) ;
#68988=FACE_OUTER_BOUND ( 'NONE', #25643, .T. ) ;
#69001=ORIENTED_EDGE ( 'NONE', *, *, #14306, .T. ) ;
#69008=PLANE ( 'NONE',  #756 ) ;
#69036=VECTOR ( 'NONE', #43678, 1000.000000000000000 ) ;
#69075=AXIS2_PLACEMENT_3D ( 'NONE', #29367, #14572, #13542 ) ;
#69082=VECTOR ( 'NONE', #10347, 1000.000000000000000 ) ;
#69103=CARTESIAN_POINT ( 'NONE',  ( -452.6627218934913230, 399.9999999999997726, 113.5502958579881891 ) ) ;
#69129=ADVANCED_FACE ( 'NONE', ( #22483 ), #43920, .T. ) ;
#69134=CARTESIAN_POINT ( 'NONE',  ( -417.6627218934913230, 399.9999999999998295, 78.55029585798814651 ) ) ;
#69136=VECTOR ( 'NONE', #34255, 1000.000000000000000 ) ;
#69139=AXIS2_PLACEMENT_3D ( 'NONE', #26220, #10373, #47659 ) ;
#69155=EDGE_CURVE ( 'NONE', #62318, #28106, #50607, .T. ) ;
#69179=DIRECTION ( 'NONE',  ( -1.850371928290090422E-16, 1.000000000000000000, 1.110223024625156171E-16 ) ) ;
#69190=CARTESIAN_POINT ( 'NONE',  ( 14.83727810650406731, 400.0000000000001137, -353.9497041420119672 ) ) ;
#69194=CARTESIAN_POINT ( 'NONE',  ( -452.6627218934918346, 365.0000000000064233, -146.4497041420121377 ) ) ;
#69224=CARTESIAN_POINT ( 'NONE',  ( 447.3372781065085633, 177.8591479523844612, -111.4497041420119388 ) ) ;
#69232=AXIS2_PLACEMENT_3D ( 'NONE', #56206, #30871, #25253 ) ;
#69235=EDGE_CURVE ( 'NONE', #7387, #12094, #61514, .T. ) ;
#69260=CARTESIAN_POINT ( 'NONE',  ( -452.6627218934859798, 400.0000000000066507, -146.4497041420121377 ) ) ;
#69263=SURFACE_STYLE_FILL_AREA ( #54808 ) ;
#69284=DIRECTION ( 'NONE',  ( -3.049318610115480619E-20, -1.000000000000000000, -6.106226635438359986E-16 ) ) ;
#69285=ORIENTED_EDGE ( 'NONE', *, *, #15489, .F. ) ;
#69291=PLANE ( 'NONE',  #8068 ) ;
#69299=DIRECTION ( 'NONE',  ( -1.387778780781445429E-16, 1.000000000000000000, 3.081487911019577365E-33 ) ) ;
#69311=DIRECTION ( 'NONE',  ( 1.000000000000000000, 6.405132834375897126E-16, 4.102572662600025274E-31 ) ) ;
#69312=DIRECTION ( 'NONE',  ( 0.000000000000000000, -3.469446951953614805E-17, 1.000000000000000000 ) ) ;
#69332=VECTOR ( 'NONE', #12391, 1000.000000000000114 ) ;
#69333=CARTESIAN_POINT ( 'NONE',  ( -443.8104064242511981, 394.8690347851185152, 98.47546630130500489 ) ) ;
#69363=( LENGTH_UNIT ( ) NAMED_UNIT ( * ) SI_UNIT ( .MILLI., .METRE. ) );
#69386=PLANE ( 'NONE',  #59861 ) ;
#69426=ORIENTED_EDGE ( 'NONE', *, *, #63160, .F. ) ;
#69437=ORIENTED_EDGE ( 'NONE', *, *, #18818, .T. ) ;
#69461=DIRECTION ( 'NONE',  ( 1.387778780781445922E-16, -1.000000000000000000, -1.232595164407830946E-32 ) ) ;
#69466=EDGE_CURVE ( 'NONE', #66593, #63326, #65711, .T. ) ;
#69475=ORIENTED_EDGE ( 'NONE', *, *, #26188, .F. ) ;
#69492=ORIENTED_EDGE ( 'NONE', *, *, #35651, .F. ) ;
#69501=CARTESIAN_POINT ( 'NONE',  ( 433.3728120124415568, 400.0000000000067075, -132.4852380479447902 ) ) ;
#69502=DIRECTION ( 'NONE',  ( 1.000000000000000000, 0.000000000000000000, 0.000000000000000000 ) ) ;
#69547=EDGE_CURVE ( 'NONE', #6104, #34219, #32953, .T. ) ;
#69550=EDGE_CURVE ( 'NONE', #64521, #68286, #56714, .T. ) ;
#69561=ADVANCED_FACE ( 'NONE', ( #59333 ), #11146, .T. ) ;
ENDSEC;
END-ISO-10303-21;
